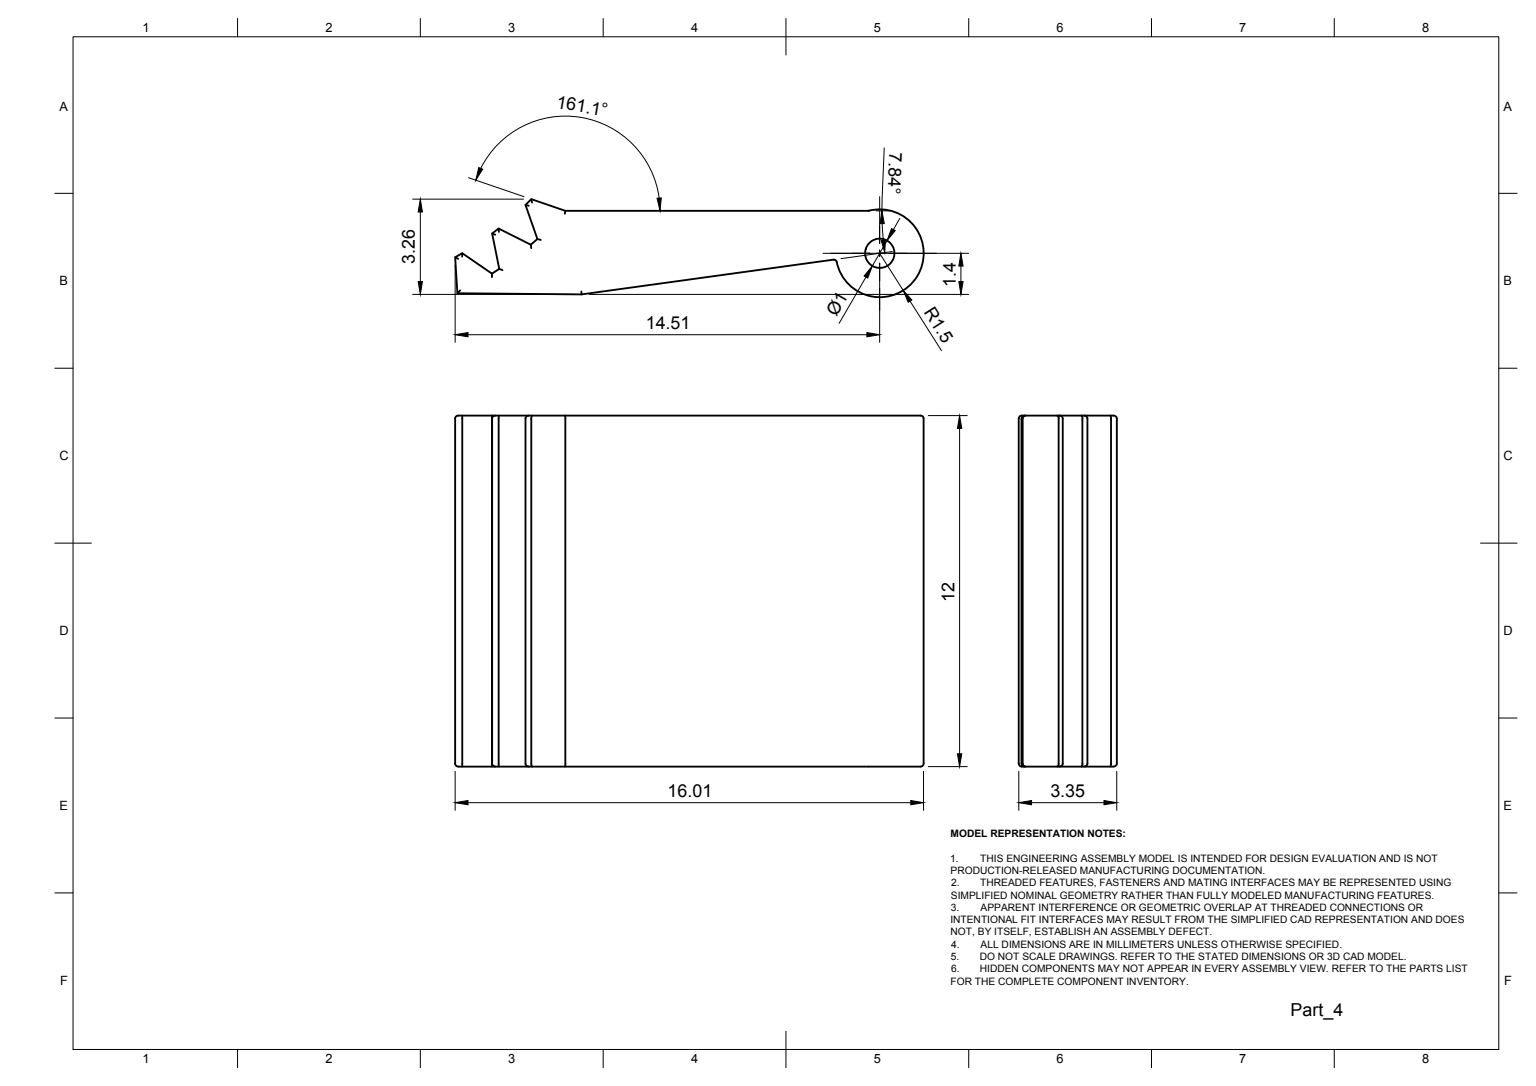
ISO-10303-21;
HEADER;
/* Generated by software containing ST-Developer
 * from STEP Tools, Inc. (www.steptools.com) 
 */

FILE_DESCRIPTION(
/* description */ ('STEP AP242 Edition 2'),
/* implementation_level */ '2;1');

FILE_NAME(
/* name */ 'Part_4.step',
/* time_stamp */ '2026-10-06T10:11:12-07:00',
/* author */ (''),
/* organization */ (''),
/* preprocessor_version */ 'ST-DEVELOPER v20.2',
/* originating_system */ 'Autodesk Translation Framework v15.15.0.0',
/* authorisation */ '');

FILE_SCHEMA (('AUTOMOTIVE_DESIGN { 1 0 10303 214 3 1 1 }'));
ENDSEC;

DATA;
#10=MECHANICAL_DESIGN_GEOMETRIC_PRESENTATION_REPRESENTATION('',(#1792),#54580);
#72=ELLIPSE('',#18845,0.000117970312899575,0.0001);
#73=ELLIPSE('',#18846,0.000120617936713865,0.0001);
#74=ELLIPSE('',#18848,0.000120617936713866,0.0001);
#75=ELLIPSE('',#18850,0.000120617936713866,0.0001);
#76=ELLIPSE('',#18851,0.000120617936713865,0.0001);
#77=ELLIPSE('',#18853,0.000117970312899575,0.0001);
#78=ELLIPSE('',#18855,0.000117970312899575,0.0001);
#79=ELLIPSE('',#18857,0.000117970312899574,0.0001);
#80=ELLIPSE('',#18859,0.000117970312899574,0.0001);
#81=ELLIPSE('',#18861,0.000117970312899575,0.0001);
#82=ELLIPSE('',#18863,0.000120617936713865,0.0001);
#83=ELLIPSE('',#18865,0.000117970312899575,0.0001);
#84=ELLIPSE('',#18867,0.000117970312899575,0.0001);
#85=ELLIPSE('',#18869,0.000120617936713865,0.0001);
#86=ELLIPSE('',#18871,0.000120617936713865,0.0001);
#87=ELLIPSE('',#18873,0.000136567519156022,0.0001);
#88=ELLIPSE('',#18875,0.000136567519156022,0.0001);
#89=ELLIPSE('',#18877,0.000120617936713865,0.0001);
#90=ELLIPSE('',#18879,0.000117970312899574,0.0001);
#91=ELLIPSE('',#18881,0.000100268099705458,0.0001);
#92=ELLIPSE('',#18883,0.000100268099705458,0.0001);
#93=ELLIPSE('',#18885,0.000117970312899574,0.0001);
#94=ELLIPSE('',#18887,0.000117970312899575,0.0001);
#95=ELLIPSE('',#18896,0.000117970312899575,0.0001);
#96=ELLIPSE('',#18898,0.000101375812252276,0.0001);
#97=ELLIPSE('',#18904,0.000101375812252276,0.0001);
#240=TOROIDAL_SURFACE('',#18899,0.0002,0.0001);
#241=TOROIDAL_SURFACE('',#18901,0.0002,0.0001);
#242=TOROIDAL_SURFACE('',#18907,0.0014,0.0001);
#243=TOROIDAL_SURFACE('',#18909,0.0014,0.0001);
#244=TOROIDAL_SURFACE('',#18913,0.0002,0.0001);
#245=TOROIDAL_SURFACE('',#18915,0.0002,0.0001);
#246=TOROIDAL_SURFACE('',#18918,0.0006,0.0001);
#247=TOROIDAL_SURFACE('',#18920,0.0006,0.0001);
#1748=SHAPE_REPRESENTATION_RELATIONSHIP('SRR','None',#54635,#1762);
#1762=ADVANCED_BREP_SHAPE_REPRESENTATION('',(#1806),#54571);
#1792=STYLED_ITEM('',(#54716),#1806);
#1806=MANIFOLD_SOLID_BREP('Body1',#17671);
#2101=LINE('',#47988,#2694);
#2102=LINE('',#47990,#2695);
#2103=LINE('',#47992,#2696);
#2104=LINE('',#47994,#2697);
#2105=LINE('',#47996,#2698);
#2106=LINE('',#47998,#2699);
#2107=LINE('',#48000,#2700);
#2108=LINE('',#48002,#2701);
#2109=LINE('',#48004,#2702);
#2110=LINE('',#48012,#2703);
#2111=LINE('',#48014,#2704);
#2112=LINE('',#48016,#2705);
#2113=LINE('',#48018,#2706);
#2114=LINE('',#48019,#2707);
#2115=LINE('',#48025,#2708);
#2116=LINE('',#48027,#2709);
#2117=LINE('',#48029,#2710);
#2118=LINE('',#48031,#2711);
#2119=LINE('',#48033,#2712);
#2120=LINE('',#48035,#2713);
#2121=LINE('',#48037,#2714);
#2122=LINE('',#48039,#2715);
#2123=LINE('',#48041,#2716);
#2124=LINE('',#48043,#2717);
#2125=LINE('',#48045,#2718);
#2126=LINE('',#48047,#2719);
#2127=LINE('',#48049,#2720);
#2128=LINE('',#48051,#2721);
#2129=LINE('',#48062,#2722);
#2130=LINE('',#48064,#2723);
#2131=LINE('',#48066,#2724);
#2132=LINE('',#48067,#2725);
#2133=LINE('',#48071,#2726);
#2134=LINE('',#48072,#2727);
#2135=LINE('',#48073,#2728);
#2136=LINE('',#48077,#2729);
#2137=LINE('',#48078,#2730);
#2138=LINE('',#48079,#2731);
#2139=LINE('',#48083,#2732);
#2140=LINE('',#48084,#2733);
#2141=LINE('',#48085,#2734);
#2142=LINE('',#48089,#2735);
#2143=LINE('',#48090,#2736);
#2144=LINE('',#48091,#2737);
#2145=LINE('',#48095,#2738);
#2146=LINE('',#48096,#2739);
#2147=LINE('',#48097,#2740);
#2148=LINE('',#48101,#2741);
#2149=LINE('',#48102,#2742);
#2150=LINE('',#48103,#2743);
#2151=LINE('',#48107,#2744);
#2152=LINE('',#48108,#2745);
#2153=LINE('',#48109,#2746);
#2154=LINE('',#48113,#2747);
#2155=LINE('',#48114,#2748);
#2156=LINE('',#48115,#2749);
#2157=LINE('',#48119,#2750);
#2158=LINE('',#48123,#2751);
#2159=LINE('',#48128,#2752);
#2160=LINE('',#48130,#2753);
#2161=LINE('',#48132,#2754);
#2162=LINE('',#48133,#2755);
#2163=LINE('',#48137,#2756);
#2164=LINE('',#48138,#2757);
#2165=LINE('',#48139,#2758);
#2166=LINE('',#48143,#2759);
#2167=LINE('',#48144,#2760);
#2168=LINE('',#48145,#2761);
#2169=LINE('',#48149,#2762);
#2170=LINE('',#48150,#2763);
#2171=LINE('',#48151,#2764);
#2172=LINE('',#48153,#2765);
#2173=LINE('',#48154,#2766);
#2174=LINE('',#48161,#2767);
#2694=VECTOR('',#21845,0.999999999999999);
#2695=VECTOR('',#21846,1.);
#2696=VECTOR('',#21847,1.);
#2697=VECTOR('',#21848,1.);
#2698=VECTOR('',#21849,1.);
#2699=VECTOR('',#21850,1.);
#2700=VECTOR('',#21851,1.);
#2701=VECTOR('',#21852,1.);
#2702=VECTOR('',#21853,1.);
#2703=VECTOR('',#21860,1.);
#2704=VECTOR('',#21861,1.);
#2705=VECTOR('',#21862,1.);
#2706=VECTOR('',#21863,1.);
#2707=VECTOR('',#21864,1.);
#2708=VECTOR('',#21869,1.);
#2709=VECTOR('',#21870,1.);
#2710=VECTOR('',#21871,1.);
#2711=VECTOR('',#21872,1.);
#2712=VECTOR('',#21873,1.);
#2713=VECTOR('',#21874,1.);
#2714=VECTOR('',#21875,1.);
#2715=VECTOR('',#21876,1.);
#2716=VECTOR('',#21877,0.999999999999999);
#2717=VECTOR('',#21878,1.);
#2718=VECTOR('',#21879,1.);
#2719=VECTOR('',#21880,1.);
#2720=VECTOR('',#21881,1.);
#2721=VECTOR('',#21882,1.);
#2722=VECTOR('',#21893,1.);
#2723=VECTOR('',#21894,1.);
#2724=VECTOR('',#21895,1.);
#2725=VECTOR('',#21896,1.);
#2726=VECTOR('',#21899,1.);
#2727=VECTOR('',#21900,1.);
#2728=VECTOR('',#21901,1.);
#2729=VECTOR('',#21904,1.);
#2730=VECTOR('',#21905,1.);
#2731=VECTOR('',#21906,1.);
#2732=VECTOR('',#21909,1.);
#2733=VECTOR('',#21910,0.999999999999999);
#2734=VECTOR('',#21911,0.999999999999999);
#2735=VECTOR('',#21914,1.);
#2736=VECTOR('',#21915,1.);
#2737=VECTOR('',#21916,1.);
#2738=VECTOR('',#21919,1.);
#2739=VECTOR('',#21920,1.);
#2740=VECTOR('',#21921,1.);
#2741=VECTOR('',#21924,1.);
#2742=VECTOR('',#21925,1.);
#2743=VECTOR('',#21926,1.);
#2744=VECTOR('',#21929,1.);
#2745=VECTOR('',#21930,1.);
#2746=VECTOR('',#21931,1.);
#2747=VECTOR('',#21934,1.);
#2748=VECTOR('',#21935,1.);
#2749=VECTOR('',#21936,1.);
#2750=VECTOR('',#21939,1.);
#2751=VECTOR('',#21942,1.);
#2752=VECTOR('',#21947,1.);
#2753=VECTOR('',#21948,1.);
#2754=VECTOR('',#21949,1.);
#2755=VECTOR('',#21950,1.);
#2756=VECTOR('',#21953,1.);
#2757=VECTOR('',#21954,1.);
#2758=VECTOR('',#21955,1.);
#2759=VECTOR('',#21958,1.);
#2760=VECTOR('',#21959,1.);
#2761=VECTOR('',#21960,1.);
#2762=VECTOR('',#21963,1.);
#2763=VECTOR('',#21964,1.);
#2764=VECTOR('',#21965,1.);
#2765=VECTOR('',#21968,1.);
#2766=VECTOR('',#21969,1.);
#2767=VECTOR('',#21976,0.0005);
#3329=CYLINDRICAL_SURFACE('',#18832,0.0015);
#3330=CYLINDRICAL_SURFACE('',#18840,0.0005);
#3331=CYLINDRICAL_SURFACE('',#18844,0.0001);
#3332=CYLINDRICAL_SURFACE('',#18847,0.0001);
#3333=CYLINDRICAL_SURFACE('',#18849,0.0001);
#3334=CYLINDRICAL_SURFACE('',#18852,0.0001);
#3335=CYLINDRICAL_SURFACE('',#18854,0.0001);
#3336=CYLINDRICAL_SURFACE('',#18856,0.0001);
#3337=CYLINDRICAL_SURFACE('',#18858,0.0001);
#3338=CYLINDRICAL_SURFACE('',#18860,0.0001);
#3339=CYLINDRICAL_SURFACE('',#18862,0.0001);
#3340=CYLINDRICAL_SURFACE('',#18864,0.0001);
#3341=CYLINDRICAL_SURFACE('',#18866,0.0001);
#3342=CYLINDRICAL_SURFACE('',#18868,0.0001);
#3343=CYLINDRICAL_SURFACE('',#18870,0.0001);
#3344=CYLINDRICAL_SURFACE('',#18872,0.0001);
#3345=CYLINDRICAL_SURFACE('',#18874,0.0001);
#3346=CYLINDRICAL_SURFACE('',#18876,0.0001);
#3347=CYLINDRICAL_SURFACE('',#18878,0.0001);
#3348=CYLINDRICAL_SURFACE('',#18880,0.0001);
#3349=CYLINDRICAL_SURFACE('',#18882,0.0001);
#3350=CYLINDRICAL_SURFACE('',#18884,0.0001);
#3351=CYLINDRICAL_SURFACE('',#18886,0.0001);
#3352=CYLINDRICAL_SURFACE('',#18888,0.0001);
#3353=CYLINDRICAL_SURFACE('',#18890,0.0001);
#3354=CYLINDRICAL_SURFACE('',#18893,0.0001);
#3355=CYLINDRICAL_SURFACE('',#18895,0.0001);
#3356=CYLINDRICAL_SURFACE('',#18897,0.0001);
#3357=CYLINDRICAL_SURFACE('',#18903,0.0001);
#3358=CYLINDRICAL_SURFACE('',#18905,0.0001);
#3359=CYLINDRICAL_SURFACE('',#18911,0.0001);
#3360=CYLINDRICAL_SURFACE('',#18917,0.0001);
#3506=FACE_BOUND('',#5205,.T.);
#3507=FACE_BOUND('',#5207,.T.);
#4169=FACE_OUTER_BOUND('',#5204,.T.);
#4170=FACE_OUTER_BOUND('',#5206,.T.);
#4171=FACE_OUTER_BOUND('',#5208,.T.);
#4172=FACE_OUTER_BOUND('',#5209,.T.);
#4173=FACE_OUTER_BOUND('',#5210,.T.);
#4174=FACE_OUTER_BOUND('',#5211,.T.);
#4175=FACE_OUTER_BOUND('',#5212,.T.);
#4176=FACE_OUTER_BOUND('',#5213,.T.);
#4177=FACE_OUTER_BOUND('',#5214,.T.);
#4178=FACE_OUTER_BOUND('',#5215,.T.);
#4179=FACE_OUTER_BOUND('',#5216,.T.);
#4180=FACE_OUTER_BOUND('',#5217,.T.);
#4181=FACE_OUTER_BOUND('',#5218,.T.);
#4182=FACE_OUTER_BOUND('',#5219,.T.);
#4183=FACE_OUTER_BOUND('',#5220,.T.);
#4184=FACE_OUTER_BOUND('',#5221,.T.);
#4185=FACE_OUTER_BOUND('',#5222,.T.);
#4186=FACE_OUTER_BOUND('',#5223,.T.);
#4187=FACE_OUTER_BOUND('',#5224,.T.);
#4188=FACE_OUTER_BOUND('',#5225,.T.);
#4189=FACE_OUTER_BOUND('',#5226,.T.);
#4190=FACE_OUTER_BOUND('',#5227,.T.);
#4191=FACE_OUTER_BOUND('',#5228,.T.);
#4192=FACE_OUTER_BOUND('',#5229,.T.);
#4193=FACE_OUTER_BOUND('',#5230,.T.);
#4194=FACE_OUTER_BOUND('',#5231,.T.);
#4195=FACE_OUTER_BOUND('',#5232,.T.);
#4196=FACE_OUTER_BOUND('',#5233,.T.);
#4197=FACE_OUTER_BOUND('',#5234,.T.);
#4198=FACE_OUTER_BOUND('',#5235,.T.);
#4199=FACE_OUTER_BOUND('',#5236,.T.);
#4200=FACE_OUTER_BOUND('',#5237,.T.);
#4201=FACE_OUTER_BOUND('',#5238,.T.);
#4202=FACE_OUTER_BOUND('',#5239,.T.);
#4203=FACE_OUTER_BOUND('',#5240,.T.);
#4204=FACE_OUTER_BOUND('',#5241,.T.);
#4205=FACE_OUTER_BOUND('',#5242,.T.);
#4206=FACE_OUTER_BOUND('',#5243,.T.);
#4207=FACE_OUTER_BOUND('',#5244,.T.);
#4208=FACE_OUTER_BOUND('',#5245,.T.);
#4209=FACE_OUTER_BOUND('',#5246,.T.);
#4210=FACE_OUTER_BOUND('',#5247,.T.);
#4211=FACE_OUTER_BOUND('',#5248,.T.);
#4212=FACE_OUTER_BOUND('',#5249,.T.);
#4213=FACE_OUTER_BOUND('',#5250,.T.);
#4214=FACE_OUTER_BOUND('',#5251,.T.);
#4215=FACE_OUTER_BOUND('',#5252,.T.);
#4216=FACE_OUTER_BOUND('',#5253,.T.);
#4217=FACE_OUTER_BOUND('',#5254,.T.);
#4218=FACE_OUTER_BOUND('',#5255,.T.);
#4219=FACE_OUTER_BOUND('',#5256,.T.);
#4220=FACE_OUTER_BOUND('',#5257,.T.);
#4221=FACE_OUTER_BOUND('',#5258,.T.);
#4222=FACE_OUTER_BOUND('',#5259,.T.);
#4223=FACE_OUTER_BOUND('',#5260,.T.);
#4224=FACE_OUTER_BOUND('',#5261,.T.);
#5204=EDGE_LOOP('',(#14741,#14742,#14743,#14744,#14745,#14746,#14747,#14748,
#14749,#14750,#14751,#14752,#14753,#14754,#14755,#14756,#14757));
#5205=EDGE_LOOP('',(#14758));
#5206=EDGE_LOOP('',(#14759,#14760,#14761,#14762,#14763,#14764,#14765,#14766,
#14767,#14768,#14769,#14770,#14771,#14772,#14773,#14774,#14775));
#5207=EDGE_LOOP('',(#14776));
#5208=EDGE_LOOP('',(#14777,#14778,#14779,#14780));
#5209=EDGE_LOOP('',(#14781,#14782,#14783,#14784));
#5210=EDGE_LOOP('',(#14785,#14786,#14787,#14788));
#5211=EDGE_LOOP('',(#14789,#14790,#14791,#14792));
#5212=EDGE_LOOP('',(#14793,#14794,#14795,#14796));
#5213=EDGE_LOOP('',(#14797,#14798,#14799,#14800));
#5214=EDGE_LOOP('',(#14801,#14802,#14803,#14804));
#5215=EDGE_LOOP('',(#14805,#14806,#14807,#14808));
#5216=EDGE_LOOP('',(#14809,#14810,#14811,#14812));
#5217=EDGE_LOOP('',(#14813,#14814,#14815,#14816));
#5218=EDGE_LOOP('',(#14817,#14818,#14819,#14820));
#5219=EDGE_LOOP('',(#14821,#14822,#14823,#14824));
#5220=EDGE_LOOP('',(#14825,#14826,#14827,#14828));
#5221=EDGE_LOOP('',(#14829,#14830,#14831,#14832));
#5222=EDGE_LOOP('',(#14833,#14834,#14835,#14836));
#5223=EDGE_LOOP('',(#14837,#14838,#14839,#14840,#14841));
#5224=EDGE_LOOP('',(#14842,#14843,#14844,#14845));
#5225=EDGE_LOOP('',(#14846,#14847,#14848,#14849));
#5226=EDGE_LOOP('',(#14850,#14851,#14852,#14853));
#5227=EDGE_LOOP('',(#14854,#14855,#14856,#14857));
#5228=EDGE_LOOP('',(#14858,#14859,#14860,#14861));
#5229=EDGE_LOOP('',(#14862,#14863,#14864,#14865));
#5230=EDGE_LOOP('',(#14866,#14867,#14868,#14869));
#5231=EDGE_LOOP('',(#14870,#14871,#14872,#14873));
#5232=EDGE_LOOP('',(#14874,#14875,#14876,#14877));
#5233=EDGE_LOOP('',(#14878,#14879,#14880,#14881));
#5234=EDGE_LOOP('',(#14882,#14883,#14884,#14885));
#5235=EDGE_LOOP('',(#14886,#14887,#14888,#14889));
#5236=EDGE_LOOP('',(#14890,#14891,#14892,#14893));
#5237=EDGE_LOOP('',(#14894,#14895,#14896,#14897));
#5238=EDGE_LOOP('',(#14898,#14899,#14900,#14901));
#5239=EDGE_LOOP('',(#14902,#14903,#14904,#14905));
#5240=EDGE_LOOP('',(#14906,#14907,#14908,#14909));
#5241=EDGE_LOOP('',(#14910,#14911,#14912,#14913));
#5242=EDGE_LOOP('',(#14914,#14915,#14916,#14917));
#5243=EDGE_LOOP('',(#14918,#14919,#14920,#14921));
#5244=EDGE_LOOP('',(#14922,#14923,#14924,#14925));
#5245=EDGE_LOOP('',(#14926,#14927,#14928,#14929));
#5246=EDGE_LOOP('',(#14930,#14931,#14932,#14933));
#5247=EDGE_LOOP('',(#14934,#14935,#14936,#14937));
#5248=EDGE_LOOP('',(#14938,#14939,#14940,#14941));
#5249=EDGE_LOOP('',(#14942,#14943,#14944,#14945));
#5250=EDGE_LOOP('',(#14946,#14947,#14948,#14949));
#5251=EDGE_LOOP('',(#14950,#14951,#14952,#14953));
#5252=EDGE_LOOP('',(#14954,#14955,#14956,#14957));
#5253=EDGE_LOOP('',(#14958,#14959,#14960,#14961));
#5254=EDGE_LOOP('',(#14962,#14963,#14964,#14965));
#5255=EDGE_LOOP('',(#14966,#14967,#14968,#14969));
#5256=EDGE_LOOP('',(#14970,#14971,#14972,#14973));
#5257=EDGE_LOOP('',(#14974,#14975,#14976,#14977));
#5258=EDGE_LOOP('',(#14978,#14979,#14980,#14981));
#5259=EDGE_LOOP('',(#14982,#14983,#14984,#14985));
#5260=EDGE_LOOP('',(#14986,#14987,#14988,#14989));
#5261=EDGE_LOOP('',(#14990,#14991,#14992,#14993,#14994));
#6159=CIRCLE('',#18814,0.0002);
#6160=CIRCLE('',#18815,0.0014);
#6161=CIRCLE('',#18816,0.0002);
#6162=CIRCLE('',#18817,0.0006);
#6163=CIRCLE('',#18819,0.0002);
#6164=CIRCLE('',#18820,0.0014);
#6165=CIRCLE('',#18821,0.0002);
#6166=CIRCLE('',#18822,0.0006);
#6167=CIRCLE('',#18833,0.0015);
#6168=CIRCLE('',#18834,0.0015);
#6169=CIRCLE('',#18841,0.0005);
#6170=CIRCLE('',#18842,0.0005);
#6171=CIRCLE('',#18843,0.0005);
#6172=CIRCLE('',#18889,0.0001);
#6173=CIRCLE('',#18891,0.0001);
#6174=CIRCLE('',#18892,0.0001);
#6175=CIRCLE('',#18894,0.0001);
#6176=CIRCLE('',#18900,0.0001);
#6177=CIRCLE('',#18902,0.0001);
#6178=CIRCLE('',#18906,0.0001);
#6179=CIRCLE('',#18908,0.0001);
#6180=CIRCLE('',#18910,0.0001);
#6181=CIRCLE('',#18912,0.0001);
#6182=CIRCLE('',#18914,0.0001);
#6183=CIRCLE('',#18916,0.0001);
#6184=CIRCLE('',#18919,0.0001);
#6185=CIRCLE('',#18921,0.0001);
#7772=VERTEX_POINT('',#47986);
#7773=VERTEX_POINT('',#47987);
#7774=VERTEX_POINT('',#47989);
#7775=VERTEX_POINT('',#47991);
#7776=VERTEX_POINT('',#47993);
#7777=VERTEX_POINT('',#47995);
#7778=VERTEX_POINT('',#47997);
#7779=VERTEX_POINT('',#47999);
#7780=VERTEX_POINT('',#48001);
#7781=VERTEX_POINT('',#48003);
#7782=VERTEX_POINT('',#48005);
#7783=VERTEX_POINT('',#48007);
#7784=VERTEX_POINT('',#48009);
#7785=VERTEX_POINT('',#48011);
#7786=VERTEX_POINT('',#48013);
#7787=VERTEX_POINT('',#48015);
#7788=VERTEX_POINT('',#48017);
#7789=VERTEX_POINT('',#48020);
#7790=VERTEX_POINT('',#48023);
#7791=VERTEX_POINT('',#48024);
#7792=VERTEX_POINT('',#48026);
#7793=VERTEX_POINT('',#48028);
#7794=VERTEX_POINT('',#48030);
#7795=VERTEX_POINT('',#48032);
#7796=VERTEX_POINT('',#48034);
#7797=VERTEX_POINT('',#48036);
#7798=VERTEX_POINT('',#48038);
#7799=VERTEX_POINT('',#48040);
#7800=VERTEX_POINT('',#48042);
#7801=VERTEX_POINT('',#48044);
#7802=VERTEX_POINT('',#48046);
#7803=VERTEX_POINT('',#48048);
#7804=VERTEX_POINT('',#48050);
#7805=VERTEX_POINT('',#48052);
#7806=VERTEX_POINT('',#48054);
#7807=VERTEX_POINT('',#48057);
#7808=VERTEX_POINT('',#48060);
#7809=VERTEX_POINT('',#48061);
#7810=VERTEX_POINT('',#48063);
#7811=VERTEX_POINT('',#48065);
#7812=VERTEX_POINT('',#48069);
#7813=VERTEX_POINT('',#48070);
#7814=VERTEX_POINT('',#48075);
#7815=VERTEX_POINT('',#48076);
#7816=VERTEX_POINT('',#48081);
#7817=VERTEX_POINT('',#48082);
#7818=VERTEX_POINT('',#48087);
#7819=VERTEX_POINT('',#48088);
#7820=VERTEX_POINT('',#48093);
#7821=VERTEX_POINT('',#48094);
#7822=VERTEX_POINT('',#48099);
#7823=VERTEX_POINT('',#48100);
#7824=VERTEX_POINT('',#48105);
#7825=VERTEX_POINT('',#48106);
#7826=VERTEX_POINT('',#48111);
#7827=VERTEX_POINT('',#48112);
#7828=VERTEX_POINT('',#48117);
#7829=VERTEX_POINT('',#48118);
#7830=VERTEX_POINT('',#48120);
#7831=VERTEX_POINT('',#48122);
#7832=VERTEX_POINT('',#48126);
#7833=VERTEX_POINT('',#48127);
#7834=VERTEX_POINT('',#48129);
#7835=VERTEX_POINT('',#48131);
#7836=VERTEX_POINT('',#48135);
#7837=VERTEX_POINT('',#48136);
#7838=VERTEX_POINT('',#48141);
#7839=VERTEX_POINT('',#48142);
#7840=VERTEX_POINT('',#48147);
#7841=VERTEX_POINT('',#48148);
#7842=VERTEX_POINT('',#48156);
#7843=VERTEX_POINT('',#48157);
#7844=VERTEX_POINT('',#48160);
#10162=EDGE_CURVE('',#7772,#7773,#2101,.F.);
#10163=EDGE_CURVE('',#7773,#7774,#2102,.F.);
#10164=EDGE_CURVE('',#7774,#7775,#2103,.F.);
#10165=EDGE_CURVE('',#7775,#7776,#2104,.F.);
#10166=EDGE_CURVE('',#7776,#7777,#2105,.F.);
#10167=EDGE_CURVE('',#7777,#7778,#2106,.F.);
#10168=EDGE_CURVE('',#7778,#7779,#2107,.F.);
#10169=EDGE_CURVE('',#7779,#7780,#2108,.F.);
#10170=EDGE_CURVE('',#7780,#7781,#2109,.F.);
#10171=EDGE_CURVE('',#7782,#7781,#6159,.T.);
#10172=EDGE_CURVE('',#7782,#7783,#6160,.T.);
#10173=EDGE_CURVE('',#7784,#7783,#6161,.T.);
#10174=EDGE_CURVE('',#7784,#7785,#2110,.F.);
#10175=EDGE_CURVE('',#7785,#7786,#2111,.F.);
#10176=EDGE_CURVE('',#7786,#7787,#2112,.F.);
#10177=EDGE_CURVE('',#7787,#7788,#2113,.F.);
#10178=EDGE_CURVE('',#7788,#7772,#2114,.F.);
#10179=EDGE_CURVE('',#7789,#7789,#6162,.F.);
#10180=EDGE_CURVE('',#7790,#7791,#2115,.T.);
#10181=EDGE_CURVE('',#7791,#7792,#2116,.T.);
#10182=EDGE_CURVE('',#7792,#7793,#2117,.T.);
#10183=EDGE_CURVE('',#7793,#7794,#2118,.T.);
#10184=EDGE_CURVE('',#7794,#7795,#2119,.T.);
#10185=EDGE_CURVE('',#7795,#7796,#2120,.T.);
#10186=EDGE_CURVE('',#7796,#7797,#2121,.T.);
#10187=EDGE_CURVE('',#7797,#7798,#2122,.T.);
#10188=EDGE_CURVE('',#7798,#7799,#2123,.T.);
#10189=EDGE_CURVE('',#7799,#7800,#2124,.T.);
#10190=EDGE_CURVE('',#7800,#7801,#2125,.T.);
#10191=EDGE_CURVE('',#7801,#7802,#2126,.T.);
#10192=EDGE_CURVE('',#7802,#7803,#2127,.T.);
#10193=EDGE_CURVE('',#7803,#7804,#2128,.T.);
#10194=EDGE_CURVE('',#7805,#7804,#6163,.T.);
#10195=EDGE_CURVE('',#7805,#7806,#6164,.T.);
#10196=EDGE_CURVE('',#7790,#7806,#6165,.T.);
#10197=EDGE_CURVE('',#7807,#7807,#6166,.F.);
#10198=EDGE_CURVE('',#7808,#7809,#2129,.T.);
#10199=EDGE_CURVE('',#7809,#7810,#2130,.F.);
#10200=EDGE_CURVE('',#7811,#7810,#2131,.T.);
#10201=EDGE_CURVE('',#7811,#7808,#2132,.T.);
#10202=EDGE_CURVE('',#7812,#7813,#2133,.T.);
#10203=EDGE_CURVE('',#7813,#7809,#2134,.F.);
#10204=EDGE_CURVE('',#7808,#7812,#2135,.T.);
#10205=EDGE_CURVE('',#7814,#7815,#2136,.T.);
#10206=EDGE_CURVE('',#7815,#7813,#2137,.F.);
#10207=EDGE_CURVE('',#7812,#7814,#2138,.T.);
#10208=EDGE_CURVE('',#7816,#7817,#2139,.T.);
#10209=EDGE_CURVE('',#7817,#7815,#2140,.F.);
#10210=EDGE_CURVE('',#7814,#7816,#2141,.T.);
#10211=EDGE_CURVE('',#7818,#7819,#2142,.T.);
#10212=EDGE_CURVE('',#7819,#7817,#2143,.F.);
#10213=EDGE_CURVE('',#7816,#7818,#2144,.T.);
#10214=EDGE_CURVE('',#7820,#7821,#2145,.T.);
#10215=EDGE_CURVE('',#7821,#7819,#2146,.F.);
#10216=EDGE_CURVE('',#7818,#7820,#2147,.T.);
#10217=EDGE_CURVE('',#7822,#7823,#2148,.T.);
#10218=EDGE_CURVE('',#7823,#7821,#2149,.F.);
#10219=EDGE_CURVE('',#7820,#7822,#2150,.T.);
#10220=EDGE_CURVE('',#7824,#7825,#2151,.T.);
#10221=EDGE_CURVE('',#7825,#7823,#2152,.F.);
#10222=EDGE_CURVE('',#7822,#7824,#2153,.T.);
#10223=EDGE_CURVE('',#7826,#7827,#2154,.F.);
#10224=EDGE_CURVE('',#7827,#7825,#2155,.F.);
#10225=EDGE_CURVE('',#7824,#7826,#2156,.T.);
#10226=EDGE_CURVE('',#7828,#7829,#2157,.T.);
#10227=EDGE_CURVE('',#7829,#7830,#6167,.F.);
#10228=EDGE_CURVE('',#7830,#7831,#2158,.F.);
#10229=EDGE_CURVE('',#7831,#7828,#6168,.F.);
#10230=EDGE_CURVE('',#7832,#7833,#2159,.T.);
#10231=EDGE_CURVE('',#7833,#7834,#2160,.F.);
#10232=EDGE_CURVE('',#7834,#7835,#2161,.T.);
#10233=EDGE_CURVE('',#7835,#7832,#2162,.T.);
#10234=EDGE_CURVE('',#7836,#7837,#2163,.T.);
#10235=EDGE_CURVE('',#7837,#7833,#2164,.F.);
#10236=EDGE_CURVE('',#7832,#7836,#2165,.T.);
#10237=EDGE_CURVE('',#7838,#7839,#2166,.T.);
#10238=EDGE_CURVE('',#7839,#7837,#2167,.F.);
#10239=EDGE_CURVE('',#7836,#7838,#2168,.T.);
#10240=EDGE_CURVE('',#7840,#7841,#2169,.T.);
#10241=EDGE_CURVE('',#7841,#7839,#2170,.F.);
#10242=EDGE_CURVE('',#7838,#7840,#2171,.T.);
#10243=EDGE_CURVE('',#7810,#7841,#2172,.F.);
#10244=EDGE_CURVE('',#7840,#7811,#2173,.T.);
#10245=EDGE_CURVE('',#7842,#7843,#6169,.T.);
#10246=EDGE_CURVE('',#7843,#7842,#6170,.T.);
#10247=EDGE_CURVE('',#7842,#7844,#2174,.T.);
#10248=EDGE_CURVE('',#7844,#7844,#6171,.T.);
#10249=EDGE_CURVE('',#7774,#7812,#72,.F.);
#10250=EDGE_CURVE('',#7814,#7773,#73,.T.);
#10251=EDGE_CURVE('',#7816,#7772,#74,.T.);
#10252=EDGE_CURVE('',#7799,#7817,#75,.T.);
#10253=EDGE_CURVE('',#7815,#7798,#76,.F.);
#10254=EDGE_CURVE('',#7813,#7797,#77,.F.);
#10255=EDGE_CURVE('',#7775,#7808,#78,.F.);
#10256=EDGE_CURVE('',#7818,#7788,#79,.T.);
#10257=EDGE_CURVE('',#7800,#7819,#80,.T.);
#10258=EDGE_CURVE('',#7809,#7796,#81,.F.);
#10259=EDGE_CURVE('',#7776,#7811,#82,.F.);
#10260=EDGE_CURVE('',#7820,#7787,#83,.T.);
#10261=EDGE_CURVE('',#7801,#7821,#84,.T.);
#10262=EDGE_CURVE('',#7810,#7795,#85,.F.);
#10263=EDGE_CURVE('',#7777,#7840,#86,.F.);
#10264=EDGE_CURVE('',#7822,#7786,#87,.T.);
#10265=EDGE_CURVE('',#7802,#7823,#88,.T.);
#10266=EDGE_CURVE('',#7841,#7794,#89,.F.);
#10267=EDGE_CURVE('',#7778,#7838,#90,.F.);
#10268=EDGE_CURVE('',#7824,#7785,#91,.T.);
#10269=EDGE_CURVE('',#7803,#7825,#92,.T.);
#10270=EDGE_CURVE('',#7839,#7793,#93,.F.);
#10271=EDGE_CURVE('',#7779,#7836,#94,.F.);
#10272=EDGE_CURVE('',#7826,#7784,#6172,.T.);
#10273=EDGE_CURVE('',#7827,#7830,#6173,.F.);
#10274=EDGE_CURVE('',#7831,#7826,#6174,.F.);
#10275=EDGE_CURVE('',#7804,#7827,#6175,.T.);
#10276=EDGE_CURVE('',#7837,#7792,#95,.F.);
#10277=EDGE_CURVE('',#7780,#7832,#96,.F.);
#10278=EDGE_CURVE('',#7831,#7783,#6176,.F.);
#10279=EDGE_CURVE('',#7805,#7830,#6177,.F.);
#10280=EDGE_CURVE('',#7833,#7791,#97,.F.);
#10281=EDGE_CURVE('',#7781,#7835,#6178,.T.);
#10282=EDGE_CURVE('',#7828,#7782,#6179,.T.);
#10283=EDGE_CURVE('',#7806,#7829,#6180,.T.);
#10284=EDGE_CURVE('',#7834,#7790,#6181,.T.);
#10285=EDGE_CURVE('',#7828,#7835,#6182,.T.);
#10286=EDGE_CURVE('',#7834,#7829,#6183,.T.);
#10287=EDGE_CURVE('',#7844,#7807,#6184,.T.);
#10288=EDGE_CURVE('',#7843,#7789,#6185,.T.);
#14741=ORIENTED_EDGE('',*,*,#10162,.T.);
#14742=ORIENTED_EDGE('',*,*,#10163,.T.);
#14743=ORIENTED_EDGE('',*,*,#10164,.T.);
#14744=ORIENTED_EDGE('',*,*,#10165,.T.);
#14745=ORIENTED_EDGE('',*,*,#10166,.T.);
#14746=ORIENTED_EDGE('',*,*,#10167,.T.);
#14747=ORIENTED_EDGE('',*,*,#10168,.T.);
#14748=ORIENTED_EDGE('',*,*,#10169,.T.);
#14749=ORIENTED_EDGE('',*,*,#10170,.T.);
#14750=ORIENTED_EDGE('',*,*,#10171,.F.);
#14751=ORIENTED_EDGE('',*,*,#10172,.T.);
#14752=ORIENTED_EDGE('',*,*,#10173,.F.);
#14753=ORIENTED_EDGE('',*,*,#10174,.T.);
#14754=ORIENTED_EDGE('',*,*,#10175,.T.);
#14755=ORIENTED_EDGE('',*,*,#10176,.T.);
#14756=ORIENTED_EDGE('',*,*,#10177,.T.);
#14757=ORIENTED_EDGE('',*,*,#10178,.T.);
#14758=ORIENTED_EDGE('',*,*,#10179,.T.);
#14759=ORIENTED_EDGE('',*,*,#10180,.T.);
#14760=ORIENTED_EDGE('',*,*,#10181,.T.);
#14761=ORIENTED_EDGE('',*,*,#10182,.T.);
#14762=ORIENTED_EDGE('',*,*,#10183,.T.);
#14763=ORIENTED_EDGE('',*,*,#10184,.T.);
#14764=ORIENTED_EDGE('',*,*,#10185,.T.);
#14765=ORIENTED_EDGE('',*,*,#10186,.T.);
#14766=ORIENTED_EDGE('',*,*,#10187,.T.);
#14767=ORIENTED_EDGE('',*,*,#10188,.T.);
#14768=ORIENTED_EDGE('',*,*,#10189,.T.);
#14769=ORIENTED_EDGE('',*,*,#10190,.T.);
#14770=ORIENTED_EDGE('',*,*,#10191,.T.);
#14771=ORIENTED_EDGE('',*,*,#10192,.T.);
#14772=ORIENTED_EDGE('',*,*,#10193,.T.);
#14773=ORIENTED_EDGE('',*,*,#10194,.F.);
#14774=ORIENTED_EDGE('',*,*,#10195,.T.);
#14775=ORIENTED_EDGE('',*,*,#10196,.F.);
#14776=ORIENTED_EDGE('',*,*,#10197,.T.);
#14777=ORIENTED_EDGE('',*,*,#10198,.T.);
#14778=ORIENTED_EDGE('',*,*,#10199,.T.);
#14779=ORIENTED_EDGE('',*,*,#10200,.F.);
#14780=ORIENTED_EDGE('',*,*,#10201,.T.);
#14781=ORIENTED_EDGE('',*,*,#10202,.T.);
#14782=ORIENTED_EDGE('',*,*,#10203,.T.);
#14783=ORIENTED_EDGE('',*,*,#10198,.F.);
#14784=ORIENTED_EDGE('',*,*,#10204,.T.);
#14785=ORIENTED_EDGE('',*,*,#10205,.T.);
#14786=ORIENTED_EDGE('',*,*,#10206,.T.);
#14787=ORIENTED_EDGE('',*,*,#10202,.F.);
#14788=ORIENTED_EDGE('',*,*,#10207,.T.);
#14789=ORIENTED_EDGE('',*,*,#10208,.T.);
#14790=ORIENTED_EDGE('',*,*,#10209,.T.);
#14791=ORIENTED_EDGE('',*,*,#10205,.F.);
#14792=ORIENTED_EDGE('',*,*,#10210,.T.);
#14793=ORIENTED_EDGE('',*,*,#10211,.T.);
#14794=ORIENTED_EDGE('',*,*,#10212,.T.);
#14795=ORIENTED_EDGE('',*,*,#10208,.F.);
#14796=ORIENTED_EDGE('',*,*,#10213,.T.);
#14797=ORIENTED_EDGE('',*,*,#10214,.T.);
#14798=ORIENTED_EDGE('',*,*,#10215,.T.);
#14799=ORIENTED_EDGE('',*,*,#10211,.F.);
#14800=ORIENTED_EDGE('',*,*,#10216,.T.);
#14801=ORIENTED_EDGE('',*,*,#10217,.T.);
#14802=ORIENTED_EDGE('',*,*,#10218,.T.);
#14803=ORIENTED_EDGE('',*,*,#10214,.F.);
#14804=ORIENTED_EDGE('',*,*,#10219,.T.);
#14805=ORIENTED_EDGE('',*,*,#10220,.T.);
#14806=ORIENTED_EDGE('',*,*,#10221,.T.);
#14807=ORIENTED_EDGE('',*,*,#10217,.F.);
#14808=ORIENTED_EDGE('',*,*,#10222,.T.);
#14809=ORIENTED_EDGE('',*,*,#10223,.T.);
#14810=ORIENTED_EDGE('',*,*,#10224,.T.);
#14811=ORIENTED_EDGE('',*,*,#10220,.F.);
#14812=ORIENTED_EDGE('',*,*,#10225,.T.);
#14813=ORIENTED_EDGE('',*,*,#10226,.T.);
#14814=ORIENTED_EDGE('',*,*,#10227,.T.);
#14815=ORIENTED_EDGE('',*,*,#10228,.T.);
#14816=ORIENTED_EDGE('',*,*,#10229,.T.);
#14817=ORIENTED_EDGE('',*,*,#10230,.T.);
#14818=ORIENTED_EDGE('',*,*,#10231,.T.);
#14819=ORIENTED_EDGE('',*,*,#10232,.T.);
#14820=ORIENTED_EDGE('',*,*,#10233,.T.);
#14821=ORIENTED_EDGE('',*,*,#10234,.T.);
#14822=ORIENTED_EDGE('',*,*,#10235,.T.);
#14823=ORIENTED_EDGE('',*,*,#10230,.F.);
#14824=ORIENTED_EDGE('',*,*,#10236,.T.);
#14825=ORIENTED_EDGE('',*,*,#10237,.T.);
#14826=ORIENTED_EDGE('',*,*,#10238,.T.);
#14827=ORIENTED_EDGE('',*,*,#10234,.F.);
#14828=ORIENTED_EDGE('',*,*,#10239,.T.);
#14829=ORIENTED_EDGE('',*,*,#10240,.T.);
#14830=ORIENTED_EDGE('',*,*,#10241,.T.);
#14831=ORIENTED_EDGE('',*,*,#10237,.F.);
#14832=ORIENTED_EDGE('',*,*,#10242,.T.);
#14833=ORIENTED_EDGE('',*,*,#10200,.T.);
#14834=ORIENTED_EDGE('',*,*,#10243,.T.);
#14835=ORIENTED_EDGE('',*,*,#10240,.F.);
#14836=ORIENTED_EDGE('',*,*,#10244,.T.);
#14837=ORIENTED_EDGE('',*,*,#10245,.T.);
#14838=ORIENTED_EDGE('',*,*,#10246,.T.);
#14839=ORIENTED_EDGE('',*,*,#10247,.T.);
#14840=ORIENTED_EDGE('',*,*,#10248,.T.);
#14841=ORIENTED_EDGE('',*,*,#10247,.F.);
#14842=ORIENTED_EDGE('',*,*,#10249,.F.);
#14843=ORIENTED_EDGE('',*,*,#10163,.F.);
#14844=ORIENTED_EDGE('',*,*,#10250,.F.);
#14845=ORIENTED_EDGE('',*,*,#10207,.F.);
#14846=ORIENTED_EDGE('',*,*,#10250,.T.);
#14847=ORIENTED_EDGE('',*,*,#10162,.F.);
#14848=ORIENTED_EDGE('',*,*,#10251,.F.);
#14849=ORIENTED_EDGE('',*,*,#10210,.F.);
#14850=ORIENTED_EDGE('',*,*,#10252,.F.);
#14851=ORIENTED_EDGE('',*,*,#10188,.F.);
#14852=ORIENTED_EDGE('',*,*,#10253,.F.);
#14853=ORIENTED_EDGE('',*,*,#10209,.F.);
#14854=ORIENTED_EDGE('',*,*,#10253,.T.);
#14855=ORIENTED_EDGE('',*,*,#10187,.F.);
#14856=ORIENTED_EDGE('',*,*,#10254,.F.);
#14857=ORIENTED_EDGE('',*,*,#10206,.F.);
#14858=ORIENTED_EDGE('',*,*,#10249,.T.);
#14859=ORIENTED_EDGE('',*,*,#10204,.F.);
#14860=ORIENTED_EDGE('',*,*,#10255,.F.);
#14861=ORIENTED_EDGE('',*,*,#10164,.F.);
#14862=ORIENTED_EDGE('',*,*,#10251,.T.);
#14863=ORIENTED_EDGE('',*,*,#10178,.F.);
#14864=ORIENTED_EDGE('',*,*,#10256,.F.);
#14865=ORIENTED_EDGE('',*,*,#10213,.F.);
#14866=ORIENTED_EDGE('',*,*,#10252,.T.);
#14867=ORIENTED_EDGE('',*,*,#10212,.F.);
#14868=ORIENTED_EDGE('',*,*,#10257,.F.);
#14869=ORIENTED_EDGE('',*,*,#10189,.F.);
#14870=ORIENTED_EDGE('',*,*,#10254,.T.);
#14871=ORIENTED_EDGE('',*,*,#10186,.F.);
#14872=ORIENTED_EDGE('',*,*,#10258,.F.);
#14873=ORIENTED_EDGE('',*,*,#10203,.F.);
#14874=ORIENTED_EDGE('',*,*,#10255,.T.);
#14875=ORIENTED_EDGE('',*,*,#10201,.F.);
#14876=ORIENTED_EDGE('',*,*,#10259,.F.);
#14877=ORIENTED_EDGE('',*,*,#10165,.F.);
#14878=ORIENTED_EDGE('',*,*,#10256,.T.);
#14879=ORIENTED_EDGE('',*,*,#10177,.F.);
#14880=ORIENTED_EDGE('',*,*,#10260,.F.);
#14881=ORIENTED_EDGE('',*,*,#10216,.F.);
#14882=ORIENTED_EDGE('',*,*,#10257,.T.);
#14883=ORIENTED_EDGE('',*,*,#10215,.F.);
#14884=ORIENTED_EDGE('',*,*,#10261,.F.);
#14885=ORIENTED_EDGE('',*,*,#10190,.F.);
#14886=ORIENTED_EDGE('',*,*,#10258,.T.);
#14887=ORIENTED_EDGE('',*,*,#10185,.F.);
#14888=ORIENTED_EDGE('',*,*,#10262,.F.);
#14889=ORIENTED_EDGE('',*,*,#10199,.F.);
#14890=ORIENTED_EDGE('',*,*,#10259,.T.);
#14891=ORIENTED_EDGE('',*,*,#10244,.F.);
#14892=ORIENTED_EDGE('',*,*,#10263,.F.);
#14893=ORIENTED_EDGE('',*,*,#10166,.F.);
#14894=ORIENTED_EDGE('',*,*,#10260,.T.);
#14895=ORIENTED_EDGE('',*,*,#10176,.F.);
#14896=ORIENTED_EDGE('',*,*,#10264,.F.);
#14897=ORIENTED_EDGE('',*,*,#10219,.F.);
#14898=ORIENTED_EDGE('',*,*,#10261,.T.);
#14899=ORIENTED_EDGE('',*,*,#10218,.F.);
#14900=ORIENTED_EDGE('',*,*,#10265,.F.);
#14901=ORIENTED_EDGE('',*,*,#10191,.F.);
#14902=ORIENTED_EDGE('',*,*,#10262,.T.);
#14903=ORIENTED_EDGE('',*,*,#10184,.F.);
#14904=ORIENTED_EDGE('',*,*,#10266,.F.);
#14905=ORIENTED_EDGE('',*,*,#10243,.F.);
#14906=ORIENTED_EDGE('',*,*,#10263,.T.);
#14907=ORIENTED_EDGE('',*,*,#10242,.F.);
#14908=ORIENTED_EDGE('',*,*,#10267,.F.);
#14909=ORIENTED_EDGE('',*,*,#10167,.F.);
#14910=ORIENTED_EDGE('',*,*,#10264,.T.);
#14911=ORIENTED_EDGE('',*,*,#10175,.F.);
#14912=ORIENTED_EDGE('',*,*,#10268,.F.);
#14913=ORIENTED_EDGE('',*,*,#10222,.F.);
#14914=ORIENTED_EDGE('',*,*,#10265,.T.);
#14915=ORIENTED_EDGE('',*,*,#10221,.F.);
#14916=ORIENTED_EDGE('',*,*,#10269,.F.);
#14917=ORIENTED_EDGE('',*,*,#10192,.F.);
#14918=ORIENTED_EDGE('',*,*,#10266,.T.);
#14919=ORIENTED_EDGE('',*,*,#10183,.F.);
#14920=ORIENTED_EDGE('',*,*,#10270,.F.);
#14921=ORIENTED_EDGE('',*,*,#10241,.F.);
#14922=ORIENTED_EDGE('',*,*,#10267,.T.);
#14923=ORIENTED_EDGE('',*,*,#10239,.F.);
#14924=ORIENTED_EDGE('',*,*,#10271,.F.);
#14925=ORIENTED_EDGE('',*,*,#10168,.F.);
#14926=ORIENTED_EDGE('',*,*,#10268,.T.);
#14927=ORIENTED_EDGE('',*,*,#10174,.F.);
#14928=ORIENTED_EDGE('',*,*,#10272,.F.);
#14929=ORIENTED_EDGE('',*,*,#10225,.F.);
#14930=ORIENTED_EDGE('',*,*,#10273,.F.);
#14931=ORIENTED_EDGE('',*,*,#10223,.F.);
#14932=ORIENTED_EDGE('',*,*,#10274,.F.);
#14933=ORIENTED_EDGE('',*,*,#10228,.F.);
#14934=ORIENTED_EDGE('',*,*,#10269,.T.);
#14935=ORIENTED_EDGE('',*,*,#10224,.F.);
#14936=ORIENTED_EDGE('',*,*,#10275,.F.);
#14937=ORIENTED_EDGE('',*,*,#10193,.F.);
#14938=ORIENTED_EDGE('',*,*,#10270,.T.);
#14939=ORIENTED_EDGE('',*,*,#10182,.F.);
#14940=ORIENTED_EDGE('',*,*,#10276,.F.);
#14941=ORIENTED_EDGE('',*,*,#10238,.F.);
#14942=ORIENTED_EDGE('',*,*,#10271,.T.);
#14943=ORIENTED_EDGE('',*,*,#10236,.F.);
#14944=ORIENTED_EDGE('',*,*,#10277,.F.);
#14945=ORIENTED_EDGE('',*,*,#10169,.F.);
#14946=ORIENTED_EDGE('',*,*,#10272,.T.);
#14947=ORIENTED_EDGE('',*,*,#10173,.T.);
#14948=ORIENTED_EDGE('',*,*,#10278,.F.);
#14949=ORIENTED_EDGE('',*,*,#10274,.T.);
#14950=ORIENTED_EDGE('',*,*,#10275,.T.);
#14951=ORIENTED_EDGE('',*,*,#10273,.T.);
#14952=ORIENTED_EDGE('',*,*,#10279,.F.);
#14953=ORIENTED_EDGE('',*,*,#10194,.T.);
#14954=ORIENTED_EDGE('',*,*,#10276,.T.);
#14955=ORIENTED_EDGE('',*,*,#10181,.F.);
#14956=ORIENTED_EDGE('',*,*,#10280,.F.);
#14957=ORIENTED_EDGE('',*,*,#10235,.F.);
#14958=ORIENTED_EDGE('',*,*,#10277,.T.);
#14959=ORIENTED_EDGE('',*,*,#10233,.F.);
#14960=ORIENTED_EDGE('',*,*,#10281,.F.);
#14961=ORIENTED_EDGE('',*,*,#10170,.F.);
#14962=ORIENTED_EDGE('',*,*,#10278,.T.);
#14963=ORIENTED_EDGE('',*,*,#10172,.F.);
#14964=ORIENTED_EDGE('',*,*,#10282,.F.);
#14965=ORIENTED_EDGE('',*,*,#10229,.F.);
#14966=ORIENTED_EDGE('',*,*,#10279,.T.);
#14967=ORIENTED_EDGE('',*,*,#10227,.F.);
#14968=ORIENTED_EDGE('',*,*,#10283,.F.);
#14969=ORIENTED_EDGE('',*,*,#10195,.F.);
#14970=ORIENTED_EDGE('',*,*,#10280,.T.);
#14971=ORIENTED_EDGE('',*,*,#10180,.F.);
#14972=ORIENTED_EDGE('',*,*,#10284,.F.);
#14973=ORIENTED_EDGE('',*,*,#10231,.F.);
#14974=ORIENTED_EDGE('',*,*,#10171,.T.);
#14975=ORIENTED_EDGE('',*,*,#10281,.T.);
#14976=ORIENTED_EDGE('',*,*,#10285,.F.);
#14977=ORIENTED_EDGE('',*,*,#10282,.T.);
#14978=ORIENTED_EDGE('',*,*,#10196,.T.);
#14979=ORIENTED_EDGE('',*,*,#10283,.T.);
#14980=ORIENTED_EDGE('',*,*,#10286,.F.);
#14981=ORIENTED_EDGE('',*,*,#10284,.T.);
#14982=ORIENTED_EDGE('',*,*,#10285,.T.);
#14983=ORIENTED_EDGE('',*,*,#10232,.F.);
#14984=ORIENTED_EDGE('',*,*,#10286,.T.);
#14985=ORIENTED_EDGE('',*,*,#10226,.F.);
#14986=ORIENTED_EDGE('',*,*,#10248,.F.);
#14987=ORIENTED_EDGE('',*,*,#10287,.T.);
#14988=ORIENTED_EDGE('',*,*,#10197,.F.);
#14989=ORIENTED_EDGE('',*,*,#10287,.F.);
#14990=ORIENTED_EDGE('',*,*,#10245,.F.);
#14991=ORIENTED_EDGE('',*,*,#10246,.F.);
#14992=ORIENTED_EDGE('',*,*,#10288,.T.);
#14993=ORIENTED_EDGE('',*,*,#10179,.F.);
#14994=ORIENTED_EDGE('',*,*,#10288,.F.);
#16575=PLANE('',#18813);
#16576=PLANE('',#18818);
#16577=PLANE('',#18823);
#16578=PLANE('',#18824);
#16579=PLANE('',#18825);
#16580=PLANE('',#18826);
#16581=PLANE('',#18827);
#16582=PLANE('',#18828);
#16583=PLANE('',#18829);
#16584=PLANE('',#18830);
#16585=PLANE('',#18831);
#16586=PLANE('',#18835);
#16587=PLANE('',#18836);
#16588=PLANE('',#18837);
#16589=PLANE('',#18838);
#16590=PLANE('',#18839);
#17285=ADVANCED_FACE('',(#4169,#3506),#16575,.T.);
#17286=ADVANCED_FACE('',(#4170,#3507),#16576,.T.);
#17287=ADVANCED_FACE('',(#4171),#16577,.T.);
#17288=ADVANCED_FACE('',(#4172),#16578,.T.);
#17289=ADVANCED_FACE('',(#4173),#16579,.T.);
#17290=ADVANCED_FACE('',(#4174),#16580,.T.);
#17291=ADVANCED_FACE('',(#4175),#16581,.T.);
#17292=ADVANCED_FACE('',(#4176),#16582,.T.);
#17293=ADVANCED_FACE('',(#4177),#16583,.T.);
#17294=ADVANCED_FACE('',(#4178),#16584,.T.);
#17295=ADVANCED_FACE('',(#4179),#16585,.T.);
#17296=ADVANCED_FACE('',(#4180),#3329,.T.);
#17297=ADVANCED_FACE('',(#4181),#16586,.T.);
#17298=ADVANCED_FACE('',(#4182),#16587,.T.);
#17299=ADVANCED_FACE('',(#4183),#16588,.T.);
#17300=ADVANCED_FACE('',(#4184),#16589,.T.);
#17301=ADVANCED_FACE('',(#4185),#16590,.T.);
#17302=ADVANCED_FACE('',(#4186),#3330,.F.);
#17303=ADVANCED_FACE('',(#4187),#3331,.T.);
#17304=ADVANCED_FACE('',(#4188),#3332,.T.);
#17305=ADVANCED_FACE('',(#4189),#3333,.T.);
#17306=ADVANCED_FACE('',(#4190),#3334,.T.);
#17307=ADVANCED_FACE('',(#4191),#3335,.T.);
#17308=ADVANCED_FACE('',(#4192),#3336,.T.);
#17309=ADVANCED_FACE('',(#4193),#3337,.T.);
#17310=ADVANCED_FACE('',(#4194),#3338,.T.);
#17311=ADVANCED_FACE('',(#4195),#3339,.T.);
#17312=ADVANCED_FACE('',(#4196),#3340,.T.);
#17313=ADVANCED_FACE('',(#4197),#3341,.T.);
#17314=ADVANCED_FACE('',(#4198),#3342,.T.);
#17315=ADVANCED_FACE('',(#4199),#3343,.T.);
#17316=ADVANCED_FACE('',(#4200),#3344,.T.);
#17317=ADVANCED_FACE('',(#4201),#3345,.T.);
#17318=ADVANCED_FACE('',(#4202),#3346,.T.);
#17319=ADVANCED_FACE('',(#4203),#3347,.T.);
#17320=ADVANCED_FACE('',(#4204),#3348,.T.);
#17321=ADVANCED_FACE('',(#4205),#3349,.T.);
#17322=ADVANCED_FACE('',(#4206),#3350,.T.);
#17323=ADVANCED_FACE('',(#4207),#3351,.T.);
#17324=ADVANCED_FACE('',(#4208),#3352,.T.);
#17325=ADVANCED_FACE('',(#4209),#3353,.F.);
#17326=ADVANCED_FACE('',(#4210),#3354,.T.);
#17327=ADVANCED_FACE('',(#4211),#3355,.T.);
#17328=ADVANCED_FACE('',(#4212),#3356,.T.);
#17329=ADVANCED_FACE('',(#4213),#240,.T.);
#17330=ADVANCED_FACE('',(#4214),#241,.T.);
#17331=ADVANCED_FACE('',(#4215),#3357,.T.);
#17332=ADVANCED_FACE('',(#4216),#3358,.T.);
#17333=ADVANCED_FACE('',(#4217),#242,.T.);
#17334=ADVANCED_FACE('',(#4218),#243,.T.);
#17335=ADVANCED_FACE('',(#4219),#3359,.T.);
#17336=ADVANCED_FACE('',(#4220),#244,.T.);
#17337=ADVANCED_FACE('',(#4221),#245,.T.);
#17338=ADVANCED_FACE('',(#4222),#3360,.F.);
#17339=ADVANCED_FACE('',(#4223),#246,.T.);
#17340=ADVANCED_FACE('',(#4224),#247,.T.);
#17671=CLOSED_SHELL('',(#17285,#17286,#17287,#17288,#17289,#17290,#17291,
#17292,#17293,#17294,#17295,#17296,#17297,#17298,#17299,#17300,#17301,#17302,
#17303,#17304,#17305,#17306,#17307,#17308,#17309,#17310,#17311,#17312,#17313,
#17314,#17315,#17316,#17317,#17318,#17319,#17320,#17321,#17322,#17323,#17324,
#17325,#17326,#17327,#17328,#17329,#17330,#17331,#17332,#17333,#17334,#17335,
#17336,#17337,#17338,#17339,#17340));
#18812=AXIS2_PLACEMENT_3D('',#47984,#21841,#21842);
#18813=AXIS2_PLACEMENT_3D('',#47985,#21843,#21844);
#18814=AXIS2_PLACEMENT_3D('',#48006,#21854,#21855);
#18815=AXIS2_PLACEMENT_3D('',#48008,#21856,#21857);
#18816=AXIS2_PLACEMENT_3D('',#48010,#21858,#21859);
#18817=AXIS2_PLACEMENT_3D('',#48021,#21865,#21866);
#18818=AXIS2_PLACEMENT_3D('',#48022,#21867,#21868);
#18819=AXIS2_PLACEMENT_3D('',#48053,#21883,#21884);
#18820=AXIS2_PLACEMENT_3D('',#48055,#21885,#21886);
#18821=AXIS2_PLACEMENT_3D('',#48056,#21887,#21888);
#18822=AXIS2_PLACEMENT_3D('',#48058,#21889,#21890);
#18823=AXIS2_PLACEMENT_3D('',#48059,#21891,#21892);
#18824=AXIS2_PLACEMENT_3D('',#48068,#21897,#21898);
#18825=AXIS2_PLACEMENT_3D('',#48074,#21902,#21903);
#18826=AXIS2_PLACEMENT_3D('',#48080,#21907,#21908);
#18827=AXIS2_PLACEMENT_3D('',#48086,#21912,#21913);
#18828=AXIS2_PLACEMENT_3D('',#48092,#21917,#21918);
#18829=AXIS2_PLACEMENT_3D('',#48098,#21922,#21923);
#18830=AXIS2_PLACEMENT_3D('',#48104,#21927,#21928);
#18831=AXIS2_PLACEMENT_3D('',#48110,#21932,#21933);
#18832=AXIS2_PLACEMENT_3D('',#48116,#21937,#21938);
#18833=AXIS2_PLACEMENT_3D('',#48121,#21940,#21941);
#18834=AXIS2_PLACEMENT_3D('',#48124,#21943,#21944);
#18835=AXIS2_PLACEMENT_3D('',#48125,#21945,#21946);
#18836=AXIS2_PLACEMENT_3D('',#48134,#21951,#21952);
#18837=AXIS2_PLACEMENT_3D('',#48140,#21956,#21957);
#18838=AXIS2_PLACEMENT_3D('',#48146,#21961,#21962);
#18839=AXIS2_PLACEMENT_3D('',#48152,#21966,#21967);
#18840=AXIS2_PLACEMENT_3D('',#48155,#21970,#21971);
#18841=AXIS2_PLACEMENT_3D('',#48158,#21972,#21973);
#18842=AXIS2_PLACEMENT_3D('',#48159,#21974,#21975);
#18843=AXIS2_PLACEMENT_3D('',#48162,#21977,#21978);
#18844=AXIS2_PLACEMENT_3D('',#48163,#21979,#21980);
#18845=AXIS2_PLACEMENT_3D('',#48164,#21981,#21982);
#18846=AXIS2_PLACEMENT_3D('',#48165,#21983,#21984);
#18847=AXIS2_PLACEMENT_3D('',#48166,#21985,#21986);
#18848=AXIS2_PLACEMENT_3D('',#48167,#21987,#21988);
#18849=AXIS2_PLACEMENT_3D('',#48168,#21989,#21990);
#18850=AXIS2_PLACEMENT_3D('',#48169,#21991,#21992);
#18851=AXIS2_PLACEMENT_3D('',#48170,#21993,#21994);
#18852=AXIS2_PLACEMENT_3D('',#48171,#21995,#21996);
#18853=AXIS2_PLACEMENT_3D('',#48172,#21997,#21998);
#18854=AXIS2_PLACEMENT_3D('',#48173,#21999,#22000);
#18855=AXIS2_PLACEMENT_3D('',#48174,#22001,#22002);
#18856=AXIS2_PLACEMENT_3D('',#48175,#22003,#22004);
#18857=AXIS2_PLACEMENT_3D('',#48176,#22005,#22006);
#18858=AXIS2_PLACEMENT_3D('',#48177,#22007,#22008);
#18859=AXIS2_PLACEMENT_3D('',#48178,#22009,#22010);
#18860=AXIS2_PLACEMENT_3D('',#48179,#22011,#22012);
#18861=AXIS2_PLACEMENT_3D('',#48180,#22013,#22014);
#18862=AXIS2_PLACEMENT_3D('',#48181,#22015,#22016);
#18863=AXIS2_PLACEMENT_3D('',#48182,#22017,#22018);
#18864=AXIS2_PLACEMENT_3D('',#48183,#22019,#22020);
#18865=AXIS2_PLACEMENT_3D('',#48184,#22021,#22022);
#18866=AXIS2_PLACEMENT_3D('',#48185,#22023,#22024);
#18867=AXIS2_PLACEMENT_3D('',#48186,#22025,#22026);
#18868=AXIS2_PLACEMENT_3D('',#48187,#22027,#22028);
#18869=AXIS2_PLACEMENT_3D('',#48188,#22029,#22030);
#18870=AXIS2_PLACEMENT_3D('',#48189,#22031,#22032);
#18871=AXIS2_PLACEMENT_3D('',#48190,#22033,#22034);
#18872=AXIS2_PLACEMENT_3D('',#48191,#22035,#22036);
#18873=AXIS2_PLACEMENT_3D('',#48192,#22037,#22038);
#18874=AXIS2_PLACEMENT_3D('',#48193,#22039,#22040);
#18875=AXIS2_PLACEMENT_3D('',#48194,#22041,#22042);
#18876=AXIS2_PLACEMENT_3D('',#48195,#22043,#22044);
#18877=AXIS2_PLACEMENT_3D('',#48196,#22045,#22046);
#18878=AXIS2_PLACEMENT_3D('',#48197,#22047,#22048);
#18879=AXIS2_PLACEMENT_3D('',#48198,#22049,#22050);
#18880=AXIS2_PLACEMENT_3D('',#48199,#22051,#22052);
#18881=AXIS2_PLACEMENT_3D('',#48200,#22053,#22054);
#18882=AXIS2_PLACEMENT_3D('',#48201,#22055,#22056);
#18883=AXIS2_PLACEMENT_3D('',#48202,#22057,#22058);
#18884=AXIS2_PLACEMENT_3D('',#48203,#22059,#22060);
#18885=AXIS2_PLACEMENT_3D('',#48204,#22061,#22062);
#18886=AXIS2_PLACEMENT_3D('',#48205,#22063,#22064);
#18887=AXIS2_PLACEMENT_3D('',#48206,#22065,#22066);
#18888=AXIS2_PLACEMENT_3D('',#48207,#22067,#22068);
#18889=AXIS2_PLACEMENT_3D('',#48208,#22069,#22070);
#18890=AXIS2_PLACEMENT_3D('',#48209,#22071,#22072);
#18891=AXIS2_PLACEMENT_3D('',#48210,#22073,#22074);
#18892=AXIS2_PLACEMENT_3D('',#48211,#22075,#22076);
#18893=AXIS2_PLACEMENT_3D('',#48212,#22077,#22078);
#18894=AXIS2_PLACEMENT_3D('',#48213,#22079,#22080);
#18895=AXIS2_PLACEMENT_3D('',#48214,#22081,#22082);
#18896=AXIS2_PLACEMENT_3D('',#48215,#22083,#22084);
#18897=AXIS2_PLACEMENT_3D('',#48216,#22085,#22086);
#18898=AXIS2_PLACEMENT_3D('',#48217,#22087,#22088);
#18899=AXIS2_PLACEMENT_3D('',#48218,#22089,#22090);
#18900=AXIS2_PLACEMENT_3D('',#48219,#22091,#22092);
#18901=AXIS2_PLACEMENT_3D('',#48220,#22093,#22094);
#18902=AXIS2_PLACEMENT_3D('',#48221,#22095,#22096);
#18903=AXIS2_PLACEMENT_3D('',#48222,#22097,#22098);
#18904=AXIS2_PLACEMENT_3D('',#48223,#22099,#22100);
#18905=AXIS2_PLACEMENT_3D('',#48224,#22101,#22102);
#18906=AXIS2_PLACEMENT_3D('',#48225,#22103,#22104);
#18907=AXIS2_PLACEMENT_3D('',#48226,#22105,#22106);
#18908=AXIS2_PLACEMENT_3D('',#48227,#22107,#22108);
#18909=AXIS2_PLACEMENT_3D('',#48228,#22109,#22110);
#18910=AXIS2_PLACEMENT_3D('',#48229,#22111,#22112);
#18911=AXIS2_PLACEMENT_3D('',#48230,#22113,#22114);
#18912=AXIS2_PLACEMENT_3D('',#48231,#22115,#22116);
#18913=AXIS2_PLACEMENT_3D('',#48232,#22117,#22118);
#18914=AXIS2_PLACEMENT_3D('',#48233,#22119,#22120);
#18915=AXIS2_PLACEMENT_3D('',#48234,#22121,#22122);
#18916=AXIS2_PLACEMENT_3D('',#48235,#22123,#22124);
#18917=AXIS2_PLACEMENT_3D('',#48236,#22125,#22126);
#18918=AXIS2_PLACEMENT_3D('',#48237,#22127,#22128);
#18919=AXIS2_PLACEMENT_3D('',#48238,#22129,#22130);
#18920=AXIS2_PLACEMENT_3D('',#48239,#22131,#22132);
#18921=AXIS2_PLACEMENT_3D('',#48240,#22133,#22134);
#21841=DIRECTION('axis',(0.,0.,1.));
#21842=DIRECTION('refdir',(1.,0.,0.));
#21843=DIRECTION('center_axis',(0.,1.,0.));
#21844=DIRECTION('ref_axis',(0.,0.,1.));
#21845=DIRECTION('',(0.626301308135395,0.,0.779581087140967));
#21846=DIRECTION('',(-0.488115619572884,0.,0.872778976562211));
#21847=DIRECTION('',(0.571640760429912,0.,0.82050401645276));
#21848=DIRECTION('',(0.987834679513523,0.,-0.155507703829795));
#21849=DIRECTION('',(0.514314959619115,0.,0.857601377279671));
#21850=DIRECTION('',(-0.6024126729918,0.,0.798184797787376));
#21851=DIRECTION('',(0.454591185049047,0.,0.890700204600686));
#21852=DIRECTION('',(0.999808896940505,0.,-0.0195491585141347));
#21853=DIRECTION('',(0.952234407172013,0.,0.305368030084627));
#21854=DIRECTION('center_axis',(0.,1.,0.));
#21855=DIRECTION('ref_axis',(0.,0.,1.));
#21856=DIRECTION('center_axis',(0.,1.,0.));
#21857=DIRECTION('ref_axis',(0.,0.,1.));
#21858=DIRECTION('center_axis',(0.,1.,0.));
#21859=DIRECTION('ref_axis',(0.,0.,1.));
#21860=DIRECTION('',(-0.901654311614274,0.,-0.432457515077943));
#21861=DIRECTION('',(-0.955061656436705,0.,-0.296407207072259));
#21862=DIRECTION('',(-0.364725895711544,0.,0.931114934364932));
#21863=DIRECTION('',(0.678041750029829,0.,0.735023390931532));
#21864=DIRECTION('',(0.957458971062196,0.,-0.288569434854979));
#21865=DIRECTION('center_axis',(0.,1.,0.));
#21866=DIRECTION('ref_axis',(0.,0.,1.));
#21867=DIRECTION('center_axis',(0.,-1.,0.));
#21868=DIRECTION('ref_axis',(0.,0.,-1.));
#21869=DIRECTION('',(0.952234407172013,0.,0.305368030084627));
#21870=DIRECTION('',(0.999808896940505,0.,-0.0195491585141347));
#21871=DIRECTION('',(0.454591185049047,0.,0.890700204600686));
#21872=DIRECTION('',(-0.6024126729918,0.,0.798184797787376));
#21873=DIRECTION('',(0.514314959619115,0.,0.857601377279671));
#21874=DIRECTION('',(0.987834679513523,0.,-0.155507703829795));
#21875=DIRECTION('',(0.571640760429912,0.,0.82050401645276));
#21876=DIRECTION('',(-0.488115619572884,0.,0.872778976562211));
#21877=DIRECTION('',(0.626301308135395,0.,0.779581087140967));
#21878=DIRECTION('',(0.957458971062196,0.,-0.288569434854979));
#21879=DIRECTION('',(0.678041750029829,0.,0.735023390931532));
#21880=DIRECTION('',(-0.364725895711544,0.,0.931114934364932));
#21881=DIRECTION('',(-0.955061656436705,0.,-0.296407207072259));
#21882=DIRECTION('',(-0.901654311614274,0.,-0.432457515077943));
#21883=DIRECTION('center_axis',(0.,-1.,0.));
#21884=DIRECTION('ref_axis',(0.,0.,-1.));
#21885=DIRECTION('center_axis',(0.,-1.,0.));
#21886=DIRECTION('ref_axis',(0.,0.,-1.));
#21887=DIRECTION('center_axis',(0.,-1.,0.));
#21888=DIRECTION('ref_axis',(0.,0.,-1.));
#21889=DIRECTION('center_axis',(0.,-1.,0.));
#21890=DIRECTION('ref_axis',(0.,0.,-1.));
#21891=DIRECTION('center_axis',(-0.155507703829795,0.,-0.987834679513523));
#21892=DIRECTION('ref_axis',(-0.987834679513523,0.,0.155507703829795));
#21893=DIRECTION('',(0.,-1.,0.));
#21894=DIRECTION('',(0.987834679513523,0.,-0.155507703829795));
#21895=DIRECTION('',(0.,-1.,0.));
#21896=DIRECTION('',(0.987834679513523,0.,-0.155507703829795));
#21897=DIRECTION('center_axis',(0.82050401645276,0.,-0.571640760429912));
#21898=DIRECTION('ref_axis',(-0.571640760429912,0.,-0.82050401645276));
#21899=DIRECTION('',(0.,-1.,0.));
#21900=DIRECTION('',(0.571640760429912,0.,0.82050401645276));
#21901=DIRECTION('',(0.571640760429912,0.,0.82050401645276));
#21902=DIRECTION('center_axis',(0.872778976562211,0.,0.488115619572884));
#21903=DIRECTION('ref_axis',(0.488115619572884,0.,-0.872778976562211));
#21904=DIRECTION('',(0.,-1.,0.));
#21905=DIRECTION('',(-0.488115619572884,0.,0.872778976562211));
#21906=DIRECTION('',(-0.488115619572884,0.,0.872778976562211));
#21907=DIRECTION('center_axis',(0.779581087140967,0.,-0.626301308135395));
#21908=DIRECTION('ref_axis',(-0.626301308135395,0.,-0.779581087140967));
#21909=DIRECTION('',(0.,-1.,0.));
#21910=DIRECTION('',(0.626301308135395,0.,0.779581087140967));
#21911=DIRECTION('',(0.626301308135395,0.,0.779581087140967));
#21912=DIRECTION('center_axis',(-0.288569434854979,0.,-0.957458971062195));
#21913=DIRECTION('ref_axis',(-0.957458971062195,0.,0.288569434854979));
#21914=DIRECTION('',(0.,-1.,0.));
#21915=DIRECTION('',(0.957458971062196,0.,-0.288569434854979));
#21916=DIRECTION('',(0.957458971062196,0.,-0.288569434854979));
#21917=DIRECTION('center_axis',(0.735023390931532,0.,-0.678041750029829));
#21918=DIRECTION('ref_axis',(-0.678041750029829,0.,-0.735023390931532));
#21919=DIRECTION('',(0.,-1.,0.));
#21920=DIRECTION('',(0.678041750029829,0.,0.735023390931532));
#21921=DIRECTION('',(0.678041750029829,0.,0.735023390931532));
#21922=DIRECTION('center_axis',(0.931114934364932,0.,0.364725895711544));
#21923=DIRECTION('ref_axis',(0.364725895711544,0.,-0.931114934364932));
#21924=DIRECTION('',(0.,-1.,0.));
#21925=DIRECTION('',(-0.364725895711544,0.,0.931114934364932));
#21926=DIRECTION('',(-0.364725895711544,0.,0.931114934364932));
#21927=DIRECTION('center_axis',(-0.296407207072259,0.,0.955061656436705));
#21928=DIRECTION('ref_axis',(0.955061656436705,0.,0.296407207072259));
#21929=DIRECTION('',(0.,-1.,0.));
#21930=DIRECTION('',(-0.955061656436705,0.,-0.296407207072259));
#21931=DIRECTION('',(-0.955061656436705,0.,-0.296407207072259));
#21932=DIRECTION('center_axis',(-0.432457515077943,0.,0.901654311614274));
#21933=DIRECTION('ref_axis',(0.901654311614274,0.,0.432457515077943));
#21934=DIRECTION('',(0.,1.,0.));
#21935=DIRECTION('',(-0.901654311614274,0.,-0.432457515077943));
#21936=DIRECTION('',(-0.901654311614274,0.,-0.432457515077943));
#21937=DIRECTION('center_axis',(0.,-1.,0.));
#21938=DIRECTION('ref_axis',(-0.96822474174621,0.,0.250081685595898));
#21939=DIRECTION('',(0.,-1.,0.));
#21940=DIRECTION('center_axis',(0.,-1.,0.));
#21941=DIRECTION('ref_axis',(0.,0.,-1.));
#21942=DIRECTION('',(0.,-1.,0.));
#21943=DIRECTION('center_axis',(0.,1.,0.));
#21944=DIRECTION('ref_axis',(0.,0.,1.));
#21945=DIRECTION('center_axis',(0.305368030084627,0.,-0.952234407172013));
#21946=DIRECTION('ref_axis',(-0.952234407172013,0.,-0.305368030084627));
#21947=DIRECTION('',(0.,-1.,0.));
#21948=DIRECTION('',(0.952234407172013,0.,0.305368030084627));
#21949=DIRECTION('',(0.,1.,0.));
#21950=DIRECTION('',(0.952234407172013,0.,0.305368030084627));
#21951=DIRECTION('center_axis',(-0.0195491585141347,0.,-0.999808896940505));
#21952=DIRECTION('ref_axis',(-0.999808896940505,0.,0.0195491585141347));
#21953=DIRECTION('',(0.,-1.,0.));
#21954=DIRECTION('',(0.999808896940505,0.,-0.0195491585141347));
#21955=DIRECTION('',(0.999808896940505,0.,-0.0195491585141347));
#21956=DIRECTION('center_axis',(0.890700204600685,0.,-0.454591185049047));
#21957=DIRECTION('ref_axis',(-0.454591185049047,0.,-0.890700204600686));
#21958=DIRECTION('',(0.,-1.,0.));
#21959=DIRECTION('',(0.454591185049047,0.,0.890700204600686));
#21960=DIRECTION('',(0.454591185049047,0.,0.890700204600686));
#21961=DIRECTION('center_axis',(0.798184797787376,0.,0.6024126729918));
#21962=DIRECTION('ref_axis',(0.6024126729918,0.,-0.798184797787376));
#21963=DIRECTION('',(0.,-1.,0.));
#21964=DIRECTION('',(-0.6024126729918,0.,0.798184797787376));
#21965=DIRECTION('',(-0.6024126729918,0.,0.798184797787376));
#21966=DIRECTION('center_axis',(0.857601377279671,0.,-0.514314959619115));
#21967=DIRECTION('ref_axis',(-0.514314959619115,0.,-0.857601377279671));
#21968=DIRECTION('',(0.514314959619115,0.,0.857601377279671));
#21969=DIRECTION('',(0.514314959619115,0.,0.857601377279671));
#21970=DIRECTION('center_axis',(0.,-1.,0.));
#21971=DIRECTION('ref_axis',(0.,0.,-1.));
#21972=DIRECTION('center_axis',(0.,1.,0.));
#21973=DIRECTION('ref_axis',(0.,0.,1.));
#21974=DIRECTION('center_axis',(0.,1.,0.));
#21975=DIRECTION('ref_axis',(0.,0.,1.));
#21976=DIRECTION('',(0.,-1.,0.));
#21977=DIRECTION('center_axis',(0.,-1.,0.));
#21978=DIRECTION('ref_axis',(0.,0.,-1.));
#21979=DIRECTION('center_axis',(-0.488115619572884,0.,0.872778976562211));
#21980=DIRECTION('ref_axis',(0.872778976562211,0.,0.488115619572884));
#21981=DIRECTION('center_axis',(0.0492674350094236,0.,0.998785622567522));
#21982=DIRECTION('ref_axis',(-0.998785622567522,0.,0.0492674350094236));
#21983=DIRECTION('center_axis',(0.0833383631889745,0.,0.996521307961341));
#21984=DIRECTION('ref_axis',(-0.996521307961341,0.,0.0833383631889746));
#21985=DIRECTION('center_axis',(0.626301308135395,0.,0.779581087140967));
#21986=DIRECTION('ref_axis',(0.779581087140968,0.,-0.626301308135395));
#21987=DIRECTION('center_axis',(0.955149485630946,0.,0.29612406200601));
#21988=DIRECTION('ref_axis',(-0.29612406200601,0.,0.955149485630946));
#21989=DIRECTION('center_axis',(0.626301308135395,0.,0.779581087140967));
#21990=DIRECTION('ref_axis',(0.779581087140968,0.,-0.626301308135395));
#21991=DIRECTION('center_axis',(0.955149485630946,0.,0.29612406200601));
#21992=DIRECTION('ref_axis',(0.29612406200601,0.,-0.955149485630946));
#21993=DIRECTION('center_axis',(0.0833383631889745,0.,0.996521307961341));
#21994=DIRECTION('ref_axis',(0.996521307961341,0.,-0.0833383631889746));
#21995=DIRECTION('center_axis',(-0.488115619572884,0.,0.872778976562211));
#21996=DIRECTION('ref_axis',(0.872778976562211,0.,0.488115619572884));
#21997=DIRECTION('center_axis',(0.0492674350094236,0.,0.998785622567522));
#21998=DIRECTION('ref_axis',(0.998785622567522,0.,-0.0492674350094236));
#21999=DIRECTION('center_axis',(0.571640760429912,0.,0.82050401645276));
#22000=DIRECTION('ref_axis',(0.82050401645276,0.,-0.571640760429912));
#22001=DIRECTION('center_axis',(0.919859028046646,0.,0.392249115385974));
#22002=DIRECTION('ref_axis',(-0.392249115385974,0.,0.919859028046646));
#22003=DIRECTION('center_axis',(0.957458971062196,0.,-0.288569434854979));
#22004=DIRECTION('ref_axis',(-0.288569434854979,0.,-0.957458971062195));
#22005=DIRECTION('center_axis',(0.964702659073528,0.,0.263341564468019));
#22006=DIRECTION('ref_axis',(-0.263341564468019,0.,0.964702659073528));
#22007=DIRECTION('center_axis',(0.957458971062196,0.,-0.288569434854979));
#22008=DIRECTION('ref_axis',(-0.288569434854979,0.,-0.957458971062195));
#22009=DIRECTION('center_axis',(0.964702659073528,0.,0.263341564468019));
#22010=DIRECTION('ref_axis',(0.263341564468019,0.,-0.964702659073528));
#22011=DIRECTION('center_axis',(0.571640760429912,0.,0.82050401645276));
#22012=DIRECTION('ref_axis',(0.82050401645276,0.,-0.571640760429912));
#22013=DIRECTION('center_axis',(0.919859028046646,0.,0.392249115385974));
#22014=DIRECTION('ref_axis',(0.392249115385974,0.,-0.919859028046646));
#22015=DIRECTION('center_axis',(0.987834679513523,0.,-0.155507703829795));
#22016=DIRECTION('ref_axis',(-0.155507703829795,0.,-0.987834679513523));
#22017=DIRECTION('center_axis',(0.905930950538282,0.,0.423425451356913));
#22018=DIRECTION('ref_axis',(0.423425451356913,0.,-0.905930950538282));
#22019=DIRECTION('center_axis',(0.678041750029829,0.,0.735023390931532));
#22020=DIRECTION('ref_axis',(0.735023390931532,0.,-0.678041750029829));
#22021=DIRECTION('center_axis',(0.184809846851629,0.,0.982774297845989));
#22022=DIRECTION('ref_axis',(-0.982774297845989,0.,0.184809846851629));
#22023=DIRECTION('center_axis',(0.678041750029829,0.,0.735023390931532));
#22024=DIRECTION('ref_axis',(0.735023390931532,0.,-0.678041750029829));
#22025=DIRECTION('center_axis',(0.184809846851629,0.,0.982774297845989));
#22026=DIRECTION('ref_axis',(0.982774297845989,0.,-0.184809846851629));
#22027=DIRECTION('center_axis',(0.987834679513523,0.,-0.155507703829795));
#22028=DIRECTION('ref_axis',(-0.155507703829795,0.,-0.987834679513523));
#22029=DIRECTION('center_axis',(0.905930950538282,0.,0.423425451356913));
#22030=DIRECTION('ref_axis',(0.423425451356913,0.,-0.905930950538282));
#22031=DIRECTION('center_axis',(0.514314959619115,0.,0.857601377279671));
#22032=DIRECTION('ref_axis',(0.857601377279671,0.,-0.514314959619115));
#22033=DIRECTION('center_axis',(-0.0531308220811139,0.,0.998587560379652));
#22034=DIRECTION('ref_axis',(-0.998587560379652,0.,-0.0531308220811139));
#22035=DIRECTION('center_axis',(-0.364725895711544,0.,0.931114934364932));
#22036=DIRECTION('ref_axis',(0.931114934364932,0.,0.364725895711544));
#22037=DIRECTION('center_axis',(-0.90120055904943,0.,0.433402298527587));
#22038=DIRECTION('ref_axis',(-0.433402298527587,0.,-0.90120055904943));
#22039=DIRECTION('center_axis',(-0.364725895711544,0.,0.931114934364932));
#22040=DIRECTION('ref_axis',(0.931114934364932,0.,0.364725895711544));
#22041=DIRECTION('center_axis',(-0.90120055904943,0.,0.433402298527587));
#22042=DIRECTION('ref_axis',(0.433402298527587,0.,0.90120055904943));
#22043=DIRECTION('center_axis',(0.514314959619115,0.,0.857601377279671));
#22044=DIRECTION('ref_axis',(0.857601377279671,0.,-0.514314959619115));
#22045=DIRECTION('center_axis',(-0.0531308220811139,0.,0.998587560379652));
#22046=DIRECTION('ref_axis',(-0.998587560379652,0.,-0.0531308220811139));
#22047=DIRECTION('center_axis',(-0.6024126729918,0.,0.798184797787376));
#22048=DIRECTION('ref_axis',(0.798184797787376,0.,0.6024126729918));
#22049=DIRECTION('center_axis',(-0.087192735929436,0.,0.996191460915591));
#22050=DIRECTION('ref_axis',(-0.996191460915591,0.,-0.087192735929436));
#22051=DIRECTION('center_axis',(-0.955061656436705,0.,-0.296407207072259));
#22052=DIRECTION('ref_axis',(-0.296407207072259,0.,0.955061656436705));
#22053=DIRECTION('center_axis',(-0.930846909046263,0.,-0.365409403161739));
#22054=DIRECTION('ref_axis',(0.365409403161739,0.,-0.930846909046263));
#22055=DIRECTION('center_axis',(-0.955061656436705,0.,-0.296407207072259));
#22056=DIRECTION('ref_axis',(-0.296407207072259,0.,0.955061656436705));
#22057=DIRECTION('center_axis',(-0.930846909046263,0.,-0.365409403161739));
#22058=DIRECTION('ref_axis',(-0.365409403161739,0.,0.930846909046263));
#22059=DIRECTION('center_axis',(-0.6024126729918,0.,0.798184797787376));
#22060=DIRECTION('ref_axis',(0.798184797787376,0.,0.6024126729918));
#22061=DIRECTION('center_axis',(-0.087192735929436,0.,0.996191460915591));
#22062=DIRECTION('ref_axis',(0.996191460915591,0.,0.087192735929436));
#22063=DIRECTION('center_axis',(0.454591185049047,0.,0.890700204600686));
#22064=DIRECTION('ref_axis',(0.890700204600686,0.,-0.454591185049047));
#22065=DIRECTION('center_axis',(0.857880163767375,0.,0.513849807448113));
#22066=DIRECTION('ref_axis',(-0.513849807448113,0.,0.857880163767375));
#22067=DIRECTION('center_axis',(-0.901654311614274,0.,-0.432457515077943));
#22068=DIRECTION('ref_axis',(-0.432457515077943,0.,0.901654311614274));
#22069=DIRECTION('center_axis',(-0.901654311614274,0.,-0.432457515077943));
#22070=DIRECTION('ref_axis',(-0.432457515077943,0.,0.901654311614274));
#22071=DIRECTION('center_axis',(0.,-1.,0.));
#22072=DIRECTION('ref_axis',(0.,0.,-1.));
#22073=DIRECTION('center_axis',(0.,-1.,0.));
#22074=DIRECTION('ref_axis',(0.,0.,-1.));
#22075=DIRECTION('center_axis',(0.,1.,0.));
#22076=DIRECTION('ref_axis',(0.,0.,1.));
#22077=DIRECTION('center_axis',(-0.901654311614274,0.,-0.432457515077943));
#22078=DIRECTION('ref_axis',(-0.432457515077943,0.,0.901654311614274));
#22079=DIRECTION('center_axis',(-0.901654311614274,0.,-0.432457515077943));
#22080=DIRECTION('ref_axis',(-0.432457515077943,0.,0.901654311614274));
#22081=DIRECTION('center_axis',(0.454591185049047,0.,0.890700204600686));
#22082=DIRECTION('ref_axis',(0.890700204600686,0.,-0.454591185049047));
#22083=DIRECTION('center_axis',(0.857880163767375,0.,0.513849807448113));
#22084=DIRECTION('ref_axis',(0.513849807448113,0.,-0.857880163767375));
#22085=DIRECTION('center_axis',(0.999808896940505,0.,-0.0195491585141347));
#22086=DIRECTION('ref_axis',(-0.0195491585141347,0.,-0.999808896940505));
#22087=DIRECTION('center_axis',(0.989449877530115,0.,0.144875601312438));
#22088=DIRECTION('ref_axis',(-0.144875601312438,0.,0.989449877530115));
#22089=DIRECTION('center_axis',(0.,1.,0.));
#22090=DIRECTION('ref_axis',(-0.302115636055689,0.,-0.95327128481386));
#22091=DIRECTION('center_axis',(0.48796543950748,0.,-0.872862950208262));
#22092=DIRECTION('ref_axis',(-0.872862950208263,0.,-0.48796543950748));
#22093=DIRECTION('center_axis',(0.,-1.,0.));
#22094=DIRECTION('ref_axis',(0.,0.,-1.));
#22095=DIRECTION('center_axis',(0.487965439507477,3.78543962759162E-15,
-0.872862950208264));
#22096=DIRECTION('ref_axis',(-0.872862950208264,-3.40301281036919E-32,-0.487965439507477));
#22097=DIRECTION('center_axis',(0.999808896940505,0.,-0.0195491585141347));
#22098=DIRECTION('ref_axis',(-0.0195491585141347,0.,-0.999808896940505));
#22099=DIRECTION('center_axis',(0.989449877530115,0.,0.144875601312438));
#22100=DIRECTION('ref_axis',(0.144875601312438,0.,-0.989449877530115));
#22101=DIRECTION('center_axis',(0.952234407172013,0.,0.305368030084627));
#22102=DIRECTION('ref_axis',(0.305368030084627,0.,-0.952234407172013));
#22103=DIRECTION('center_axis',(-0.952234407172012,0.,-0.30536803008463));
#22104=DIRECTION('ref_axis',(-0.30536803008463,0.,0.952234407172012));
#22105=DIRECTION('center_axis',(0.,1.,0.));
#22106=DIRECTION('ref_axis',(-0.96822474174621,0.,0.250081685595898));
#22107=DIRECTION('center_axis',(0.849631715069657,0.,0.527376477241631));
#22108=DIRECTION('ref_axis',(0.527376477241631,0.,-0.849631715069657));
#22109=DIRECTION('center_axis',(0.,-1.,0.));
#22110=DIRECTION('ref_axis',(-0.96822474174621,0.,0.250081685595898));
#22111=DIRECTION('center_axis',(0.849631715069657,0.,0.527376477241631));
#22112=DIRECTION('ref_axis',(0.527376477241631,0.,-0.849631715069657));
#22113=DIRECTION('center_axis',(0.952234407172013,0.,0.305368030084627));
#22114=DIRECTION('ref_axis',(0.305368030084627,0.,-0.952234407172013));
#22115=DIRECTION('center_axis',(-0.952234407172012,1.3243227265015E-15,
-0.30536803008463));
#22116=DIRECTION('ref_axis',(-0.30536803008463,4.13937419839926E-32,0.952234407172012));
#22117=DIRECTION('center_axis',(0.,1.,0.));
#22118=DIRECTION('ref_axis',(0.,0.,1.));
#22119=DIRECTION('center_axis',(0.,1.,0.));
#22120=DIRECTION('ref_axis',(0.,0.,1.));
#22121=DIRECTION('center_axis',(0.,-1.,0.));
#22122=DIRECTION('ref_axis',(0.,0.,-1.));
#22123=DIRECTION('center_axis',(0.,-1.,0.));
#22124=DIRECTION('ref_axis',(0.,0.,-1.));
#22125=DIRECTION('center_axis',(0.,-1.,0.));
#22126=DIRECTION('ref_axis',(0.,0.,-1.));
#22127=DIRECTION('center_axis',(0.,-1.,0.));
#22128=DIRECTION('ref_axis',(0.,0.,-1.));
#22129=DIRECTION('center_axis',(-1.,0.,0.));
#22130=DIRECTION('ref_axis',(0.,0.,1.));
#22131=DIRECTION('center_axis',(0.,1.,0.));
#22132=DIRECTION('ref_axis',(0.,0.,1.));
#22133=DIRECTION('center_axis',(-1.,0.,0.));
#22134=DIRECTION('ref_axis',(0.,0.,-1.));
#47984=CARTESIAN_POINT('',(0.,0.,0.));
#47985=CARTESIAN_POINT('Origin',(0.00625,0.013,-2.29621274840129E-18));
#47986=CARTESIAN_POINT('',(0.00310513229246118,0.013,0.00782534372202691));
#47987=CARTESIAN_POINT('',(0.00283397885998211,0.013,0.00748782871937848));
#47988=CARTESIAN_POINT('',(0.000517972272646041,0.013,0.00460500712899027));
#47989=CARTESIAN_POINT('',(0.00343760106241995,0.013,0.00640851728792926));
#47990=CARTESIAN_POINT('',(0.00683781203254235,0.013,0.000328743292588178));
#47991=CARTESIAN_POINT('',(0.00334867942190192,0.013,0.00628088369661617));
#47992=CARTESIAN_POINT('',(0.00135080799850545,0.013,0.00341324086789248));
#47993=CARTESIAN_POINT('',(0.00212708576461598,0.013,0.00647319039387763));
#47994=CARTESIAN_POINT('',(0.00714468201094909,0.013,0.00568330633008214));
#47995=CARTESIAN_POINT('',(0.00190441615676979,0.013,0.00610189696988579));
#47996=CARTESIAN_POINT('',(0.00036250172514288,0.013,0.00353081107110126));
#47997=CARTESIAN_POINT('',(0.00264938241039218,0.013,0.00511483151597876));
#47998=CARTESIAN_POINT('',(0.00641544862510175,0.013,0.000124868763181971));
#47999=CARTESIAN_POINT('',(0.00257866842927369,0.013,0.00497627854900125));
#48000=CARTESIAN_POINT('',(0.00132244326030609,0.013,0.0025149021479097));
#48001=CARTESIAN_POINT('',(0.00139305626828131,0.013,0.00499946069925261));
#48002=CARTESIAN_POINT('',(0.00634586039595321,0.013,0.00490261903953383));
#48003=CARTESIAN_POINT('',(-0.00848709681638249,0.013,0.00183103613732295));
#48004=CARTESIAN_POINT('',(0.00434333886907659,0.013,0.00594557436539644));
#48005=CARTESIAN_POINT('',(-0.00853149850581388,0.013,0.00181051559890248));
#48006=CARTESIAN_POINT('Origin',(-0.00842602321036556,0.013,0.00164058925588855));
#48007=CARTESIAN_POINT('',(-0.00804781744366059,0.013,0.00368315161531047));
#48008=CARTESIAN_POINT('Origin',(-0.00926982557395217,0.013,0.003));
#48009=CARTESIAN_POINT('',(-0.00778675335060335,0.013,0.00360041384088911));
#48010=CARTESIAN_POINT('Origin',(-0.00787324485361894,0.013,0.00378074470321196));
#48011=CARTESIAN_POINT('',(4.52079337442143E-5,0.013,0.00735683187337399));
#48012=CARTESIAN_POINT('',(0.00222095414696891,0.013,0.00840037792943047));
#48013=CARTESIAN_POINT('',(0.00400212262074066,0.013,0.00858487618139458));
#48014=CARTESIAN_POINT('',(0.0036222395132741,0.013,0.00846697793876363));
#48015=CARTESIAN_POINT('',(0.00439463505993757,0.013,0.00758282450818601));
#48016=CARTESIAN_POINT('',(0.00721658525161907,0.013,0.000378619930437244));
#48017=CARTESIAN_POINT('',(0.00428916220193663,0.013,0.00746848786485147));
#48018=CARTESIAN_POINT('',(0.00146851978854034,0.013,0.00441080277214348));
#48019=CARTESIAN_POINT('',(0.00815021035144082,0.013,0.00630480303226358));
#48020=CARTESIAN_POINT('',(-0.00926982557395217,0.013,0.0024));
#48021=CARTESIAN_POINT('Origin',(-0.00926982557395217,0.013,0.003));
#48022=CARTESIAN_POINT('Origin',(-0.00926982557395217,0.001,0.003));
#48023=CARTESIAN_POINT('',(-0.00848709681638249,0.001,0.00183103613732295));
#48024=CARTESIAN_POINT('',(0.00139305626828131,0.001,0.00499946069925261));
#48025=CARTESIAN_POINT('',(-0.00885692281820857,0.001,0.001712438198831));
#48026=CARTESIAN_POINT('',(0.00257866842927369,0.001,0.00497627854900125));
#48027=CARTESIAN_POINT('',(-0.00922667024031924,0.001,0.0052071070980081));
#48028=CARTESIAN_POINT('',(0.00264938241039218,0.001,0.00511483151597876));
#48029=CARTESIAN_POINT('',(-0.000670064127940984,0.001,-0.00138910390576812));
#48030=CARTESIAN_POINT('',(0.00190441615676979,0.001,0.00610189696988579));
#48031=CARTESIAN_POINT('',(-0.000659221951814677,0.001,0.00949866642219173));
#48032=CARTESIAN_POINT('',(0.00212708576461598,0.001,0.00647319039387763));
#48033=CARTESIAN_POINT('',(-0.00241956898424355,0.001,-0.00110819004569721));
#48034=CARTESIAN_POINT('',(0.00334867942190192,0.001,0.00628088369661617));
#48035=CARTESIAN_POINT('',(-0.00846068082425976,0.001,0.0081399462843802));
#48036=CARTESIAN_POINT('',(0.00343760106241995,0.001,0.00640851728792926));
#48037=CARTESIAN_POINT('',(-0.0023135538114868,0.001,-0.00184639733665676));
#48038=CARTESIAN_POINT('',(0.00283397885998211,0.001,0.00748782871937848));
#48039=CARTESIAN_POINT('',(0.00186205600079768,0.001,0.00922568303979271));
#48040=CARTESIAN_POINT('',(0.00310513229246119,0.001,0.00782534372202692));
#48041=CARTESIAN_POINT('',(-0.0041049730035732,0.001,-0.00114934889328565));
#48042=CARTESIAN_POINT('',(0.00428916220193663,0.001,0.00746848786485147));
#48043=CARTESIAN_POINT('',(-0.0069061235431728,0.001,0.0108426452733117));
#48044=CARTESIAN_POINT('',(0.00439463505993757,0.001,0.00758282450818601));
#48045=CARTESIAN_POINT('',(-0.00417144472326108,0.001,-0.00170313614093291));
#48046=CARTESIAN_POINT('',(0.00400212262074066,0.001,0.00858487618139458));
#48047=CARTESIAN_POINT('',(0.00413325559518032,0.001,0.00825010458353409));
#48048=CARTESIAN_POINT('',(4.52079337442122E-5,0.001,0.00735683187337399));
#48049=CARTESIAN_POINT('',(-0.00968479566385333,0.001,0.00433708631901139));
#48050=CARTESIAN_POINT('',(-0.00778675335060335,0.001,0.00360041384088911));
#48051=CARTESIAN_POINT('',(-0.00922657982244437,0.001,0.00290983456883857));
#48052=CARTESIAN_POINT('',(-0.00804781744366059,0.001,0.00368315161531047));
#48053=CARTESIAN_POINT('Origin',(-0.00787324485361894,0.001,0.00378074470321196));
#48054=CARTESIAN_POINT('',(-0.00853149850581388,0.001,0.00181051559890248));
#48055=CARTESIAN_POINT('Origin',(-0.00926982557395217,0.001,0.003));
#48056=CARTESIAN_POINT('Origin',(-0.00842602321036556,0.001,0.00164058925588855));
#48057=CARTESIAN_POINT('',(-0.00926982557395217,0.001,0.0036));
#48058=CARTESIAN_POINT('Origin',(-0.00926982557395217,0.001,0.003));
#48059=CARTESIAN_POINT('Origin',(0.00217815846891078,0.0298951219150416,
0.00636391887181847));
#48060=CARTESIAN_POINT('',(0.00339495317277858,0.0129,0.00617236763925401));
#48061=CARTESIAN_POINT('',(0.00339495317277858,0.0011,0.00617236763925401));
#48062=CARTESIAN_POINT('',(0.00339495317277858,0.0298951219150416,0.00617236763925401));
#48063=CARTESIAN_POINT('',(0.00217815846891078,0.0011,0.00636391887181847));
#48064=CARTESIAN_POINT('',(0.00217815846891078,0.0011,0.00636391887181847));
#48065=CARTESIAN_POINT('',(0.00217815846891078,0.0129,0.00636391887181847));
#48066=CARTESIAN_POINT('',(0.00217815846891078,0.0298951219150416,0.00636391887181847));
#48067=CARTESIAN_POINT('',(0.00217815846891078,0.0129,0.00636391887181847));
#48068=CARTESIAN_POINT('Origin',(0.00339495317277858,0.0298951219150416,
0.00617236763925401));
#48069=CARTESIAN_POINT('',(0.00355542811483384,0.0129,0.00640270519320544));
#48070=CARTESIAN_POINT('',(0.00355542811483384,0.0011,0.00640270519320544));
#48071=CARTESIAN_POINT('',(0.00355542811483384,0.0298951219150416,0.00640270519320544));
#48072=CARTESIAN_POINT('',(0.00339495317277858,0.0011,0.00617236763925401));
#48073=CARTESIAN_POINT('',(0.00339495317277858,0.0129,0.00617236763925401));
#48074=CARTESIAN_POINT('Origin',(0.00355542811483384,0.0298951219150416,
0.00640270519320544));
#48075=CARTESIAN_POINT('',(0.00295417720403981,0.0129,0.00747777661796151));
#48076=CARTESIAN_POINT('',(0.00295417720403981,0.0011,0.00747777661796151));
#48077=CARTESIAN_POINT('',(0.00295417720403981,0.0298951219150416,0.00747777661796151));
#48078=CARTESIAN_POINT('',(0.00355542811483384,0.0011,0.00640270519320544));
#48079=CARTESIAN_POINT('',(0.00355542811483384,0.0129,0.00640270519320544));
#48080=CARTESIAN_POINT('Origin',(0.00295417720403981,0.0298951219150416,
0.00747777661796151));
#48081=CARTESIAN_POINT('',(0.00314085016583167,0.0129,0.0077101355618168));
#48082=CARTESIAN_POINT('',(0.00314085016583167,0.0011,0.0077101355618168));
#48083=CARTESIAN_POINT('',(0.00314085016583167,0.0298951219150416,0.0077101355618168));
#48084=CARTESIAN_POINT('',(0.00295417720403981,0.0011,0.00747777661796151));
#48085=CARTESIAN_POINT('',(0.00295417720403981,0.0129,0.00747777661796151));
#48086=CARTESIAN_POINT('Origin',(0.00314085016583167,0.0298951219150416,
0.0077101355618168));
#48087=CARTESIAN_POINT('',(0.00432022868869639,0.0129,0.00735468159030551));
#48088=CARTESIAN_POINT('',(0.00432022868869639,0.0011,0.00735468159030551));
#48089=CARTESIAN_POINT('',(0.00432022868869639,0.0298951219150416,0.00735468159030551));
#48090=CARTESIAN_POINT('',(0.00314085016583167,0.0011,0.0077101355618168));
#48091=CARTESIAN_POINT('',(0.00314085016583167,0.0129,0.0077101355618168));
#48092=CARTESIAN_POINT('Origin',(0.00432022868869639,0.0298951219150416,
0.00735468159030551));
#48093=CARTESIAN_POINT('',(0.00451057325136412,0.0129,0.007561022432726));
#48094=CARTESIAN_POINT('',(0.00451057325136412,0.0011,0.007561022432726));
#48095=CARTESIAN_POINT('',(0.00451057325136412,0.0298951219150416,0.007561022432726));
#48096=CARTESIAN_POINT('',(0.00432022868869639,0.0011,0.00735468159030551));
#48097=CARTESIAN_POINT('',(0.00432022868869639,0.0129,0.00735468159030551));
#48098=CARTESIAN_POINT('Origin',(0.00451057325136412,0.0298951219150416,
0.007561022432726));
#48099=CARTESIAN_POINT('',(0.0040613112974471,0.0129,0.00870795090600599));
#48100=CARTESIAN_POINT('',(0.0040613112974471,0.0011,0.00870795090600599));
#48101=CARTESIAN_POINT('',(0.0040613112974471,0.0298951219150416,0.00870795090600599));
#48102=CARTESIAN_POINT('',(0.00451057325136412,0.0011,0.007561022432726));
#48103=CARTESIAN_POINT('',(0.00451057325136412,0.0129,0.007561022432726));
#48104=CARTESIAN_POINT('Origin',(0.0040613112974471,0.0298951219150416,
0.00870795090600599));
#48105=CARTESIAN_POINT('',(8.56902727468245E-6,0.0129,0.00745016612406076));
#48106=CARTESIAN_POINT('',(8.56902727468245E-6,0.0011,0.00745016612406076));
#48107=CARTESIAN_POINT('',(8.56902727468245E-6,0.0298951219150416,0.00745016612406076));
#48108=CARTESIAN_POINT('',(0.0040613112974471,0.0011,0.00870795090600599));
#48109=CARTESIAN_POINT('',(0.0040613112974471,0.0129,0.00870795090600599));
#48110=CARTESIAN_POINT('Origin',(8.56902727468245E-6,0.0298951219150416,
0.00745016612406076));
#48111=CARTESIAN_POINT('',(-0.00782999910211115,0.0129,0.00369057927205054));
#48112=CARTESIAN_POINT('',(-0.00782999910211115,0.0011,0.00369057927205054));
#48113=CARTESIAN_POINT('',(-0.00782999910211115,0.001,0.00369057927205053));
#48114=CARTESIAN_POINT('',(8.56902727468245E-6,0.0011,0.00745016612406076));
#48115=CARTESIAN_POINT('',(8.56902727468245E-6,0.0129,0.00745016612406076));
#48116=CARTESIAN_POINT('Origin',(-0.00926982557395217,0.0298951219150416,
0.003));
#48117=CARTESIAN_POINT('',(-0.00847876085808972,0.0129,0.00172555242739552));
#48118=CARTESIAN_POINT('',(-0.00847876085808972,0.0011,0.00172555242739552));
#48119=CARTESIAN_POINT('',(-0.00847876085808972,0.0298951219150416,0.00172555242739552));
#48120=CARTESIAN_POINT('',(-0.00796053114863977,0.0011,0.00373194815926121));
#48121=CARTESIAN_POINT('Origin',(-0.00926982557395217,0.0011,0.003));
#48122=CARTESIAN_POINT('',(-0.00796053114863977,0.0129,0.00373194815926121));
#48123=CARTESIAN_POINT('',(-0.00796053114863977,0.0298951219150416,0.00373194815926121));
#48124=CARTESIAN_POINT('Origin',(-0.00926982557395217,0.0129,0.003));
#48125=CARTESIAN_POINT('Origin',(-0.00846848477354713,0.0298951219150416,
0.00173198859563243));
#48126=CARTESIAN_POINT('',(0.0014077431500399,0.0129,0.00489915441423508));
#48127=CARTESIAN_POINT('',(0.0014077431500399,0.0011,0.00489915441423508));
#48128=CARTESIAN_POINT('',(0.0014077431500399,0.0298951219150416,0.00489915441423508));
#48129=CARTESIAN_POINT('',(-0.00845656001337402,0.0011,0.00173581269660575));
#48130=CARTESIAN_POINT('',(-0.00846848477354713,0.0011,0.00173198859563243));
#48131=CARTESIAN_POINT('',(-0.00845656001337402,0.0129,0.00173581269660575));
#48132=CARTESIAN_POINT('',(-0.00845656001337402,0.013,0.00173581269660575));
#48133=CARTESIAN_POINT('',(-0.00846848477354713,0.0129,0.00173198859563243));
#48134=CARTESIAN_POINT('Origin',(0.0014077431500399,0.0298951219150416,
0.00489915441423508));
#48135=CARTESIAN_POINT('',(0.00263928745184173,0.0129,0.00487507415765127));
#48136=CARTESIAN_POINT('',(0.00263928745184173,0.0011,0.00487507415765127));
#48137=CARTESIAN_POINT('',(0.00263928745184173,0.0298951219150416,0.00487507415765127));
#48138=CARTESIAN_POINT('',(0.0014077431500399,0.0011,0.00489915441423508));
#48139=CARTESIAN_POINT('',(0.0014077431500399,0.0129,0.00489915441423508));
#48140=CARTESIAN_POINT('Origin',(0.00263928745184173,0.0298951219150416,
0.00487507415765127));
#48141=CARTESIAN_POINT('',(0.00276690342874427,0.0129,0.00512511767031892));
#48142=CARTESIAN_POINT('',(0.00276690342874427,0.0011,0.00512511767031892));
#48143=CARTESIAN_POINT('',(0.00276690342874427,0.0298951219150416,0.00512511767031892));
#48144=CARTESIAN_POINT('',(0.00263928745184173,0.0011,0.00487507415765127));
#48145=CARTESIAN_POINT('',(0.00263928745184173,0.0129,0.00487507415765127));
#48146=CARTESIAN_POINT('Origin',(0.00276690342874427,0.0298951219150416,
0.00512511767031892));
#48147=CARTESIAN_POINT('',(0.00202486372793092,0.0129,0.00610830550002113));
#48148=CARTESIAN_POINT('',(0.00202486372793092,0.0011,0.00610830550002113));
#48149=CARTESIAN_POINT('',(0.00202486372793092,0.0298951219150416,0.00610830550002113));
#48150=CARTESIAN_POINT('',(0.00276690342874427,0.0011,0.00512511767031892));
#48151=CARTESIAN_POINT('',(0.00276690342874427,0.0129,0.00512511767031892));
#48152=CARTESIAN_POINT('Origin',(0.00202486372793092,0.0298951219150416,
0.00610830550002113));
#48153=CARTESIAN_POINT('',(0.00202486372793092,0.0011,0.00610830550002113));
#48154=CARTESIAN_POINT('',(0.00202486372793092,0.0129,0.00610830550002113));
#48155=CARTESIAN_POINT('Origin',(-0.00926982557395217,0.0172006855706717,
0.003));
#48156=CARTESIAN_POINT('',(-0.00926982557395217,0.0129,0.0035));
#48157=CARTESIAN_POINT('',(-0.00926982557395217,0.0129,0.0025));
#48158=CARTESIAN_POINT('Origin',(-0.00926982557395217,0.0129,0.003));
#48159=CARTESIAN_POINT('Origin',(-0.00926982557395217,0.0129,0.003));
#48160=CARTESIAN_POINT('',(-0.00926982557395217,0.0011,0.0035));
#48161=CARTESIAN_POINT('',(-0.00926982557395217,0.0172006855706717,0.0035));
#48162=CARTESIAN_POINT('Origin',(-0.00926982557395217,0.0011,0.003));
#48163=CARTESIAN_POINT('Origin',(0.00346815021717762,0.0129,0.00635389363124816));
#48164=CARTESIAN_POINT('Origin',(0.00343760106241995,0.0129,0.00640851728792926));
#48165=CARTESIAN_POINT('Origin',(0.00283397885998211,0.0129,0.00748782871937848));
#48166=CARTESIAN_POINT('Origin',(0.00287621909532571,0.0129,0.00754040674877505));
#48167=CARTESIAN_POINT('Origin',(0.00310513229246118,0.0129,0.00782534372202691));
#48168=CARTESIAN_POINT('Origin',(-0.0041049730035732,0.0011,-0.00114934889328566));
#48169=CARTESIAN_POINT('Origin',(0.00310513229246118,0.0011,0.00782534372202692));
#48170=CARTESIAN_POINT('Origin',(0.00283397885998211,0.0011,0.00748782871937847));
#48171=CARTESIAN_POINT('Origin',(0.00186205600079768,0.0011,0.00922568303979271));
#48172=CARTESIAN_POINT('Origin',(0.00343760106241995,0.0011,0.00640851728792926));
#48173=CARTESIAN_POINT('Origin',(0.00331290277113331,0.0129,0.006229531715297));
#48174=CARTESIAN_POINT('Origin',(0.00334867942190192,0.0129,0.00628088369661617));
#48175=CARTESIAN_POINT('Origin',(0.00316970710931718,0.0129,0.00780588145892302));
#48176=CARTESIAN_POINT('Origin',(0.00428916220193663,0.0129,0.00746848786485147));
#48177=CARTESIAN_POINT('Origin',(-0.0069061235431728,0.0011,0.0108426452733117));
#48178=CARTESIAN_POINT('Origin',(0.00428916220193663,0.0011,0.00746848786485147));
#48179=CARTESIAN_POINT('Origin',(-0.0023135538114868,0.0011,-0.00184639733665676));
#48180=CARTESIAN_POINT('Origin',(0.00334867942190192,0.0011,0.00628088369661617));
#48181=CARTESIAN_POINT('Origin',(0.00219370923929376,0.0129,0.00646270233976982));
#48182=CARTESIAN_POINT('Origin',(0.00212708576461598,0.0129,0.00647319039387763));
#48183=CARTESIAN_POINT('Origin',(0.00424672634960323,0.0129,0.00742248576530849));
#48184=CARTESIAN_POINT('Origin',(0.00439463505993757,0.0129,0.00758282450818601));
#48185=CARTESIAN_POINT('Origin',(-0.00417144472326108,0.0011,-0.00170313614093291));
#48186=CARTESIAN_POINT('Origin',(0.00439463505993757,0.0011,0.00758282450818601));
#48187=CARTESIAN_POINT('Origin',(-0.00846068082425976,0.0011,0.0081399462843802));
#48188=CARTESIAN_POINT('Origin',(0.00212708576461597,0.0011,0.00647319039387763));
#48189=CARTESIAN_POINT('Origin',(0.00193910359020296,0.0129,0.00615973699598304));
#48190=CARTESIAN_POINT('Origin',(0.00190441615676979,0.0129,0.00610189696988579));
#48191=CARTESIAN_POINT('Origin',(0.00441746175792763,0.0129,0.00752454984315485));
#48192=CARTESIAN_POINT('Origin',(0.00400212262074066,0.0129,0.00858487618139458));
#48193=CARTESIAN_POINT('Origin',(0.00413325559518032,0.0011,0.00825010458353409));
#48194=CARTESIAN_POINT('Origin',(0.00400212262074067,0.0011,0.00858487618139459));
#48195=CARTESIAN_POINT('Origin',(-0.00241956898424355,0.0011,-0.00110819004569721));
#48196=CARTESIAN_POINT('Origin',(0.00190441615676979,0.0011,0.00610189696988579));
#48197=CARTESIAN_POINT('Origin',(0.00268708494896553,0.0129,0.00506487640301974));
#48198=CARTESIAN_POINT('Origin',(0.00264938241039218,0.0129,0.00511483151597876));
#48199=CARTESIAN_POINT('Origin',(0.00409095201815432,0.0129,0.00861244474036231));
#48200=CARTESIAN_POINT('Origin',(4.52079337441844E-5,0.0129,0.00735683187337397));
#48201=CARTESIAN_POINT('Origin',(-0.00968479566385333,0.0011,0.00433708631901139));
#48202=CARTESIAN_POINT('Origin',(4.5207933744215E-5,0.0011,0.00735683187337399));
#48203=CARTESIAN_POINT('Origin',(-0.000659221951814679,0.0011,0.00949866642219173));
#48204=CARTESIAN_POINT('Origin',(0.00264938241039218,0.0011,0.00511483151597876));
#48205=CARTESIAN_POINT('Origin',(0.00255021743138166,0.0129,0.00492053327615618));
#48206=CARTESIAN_POINT('Origin',(0.00257866842927369,0.0129,0.00497627854900125));
#48207=CARTESIAN_POINT('Origin',(5.18147787824767E-5,0.0129,0.00736000069289933));
#48208=CARTESIAN_POINT('Origin',(-0.00778675335060335,0.0129,0.00360041384088911));
#48209=CARTESIAN_POINT('Origin',(-0.00787324485361894,0.0298951219150416,
0.00378074470321196));
#48210=CARTESIAN_POINT('Origin',(-0.00787324485361894,0.0011,0.00378074470321196));
#48211=CARTESIAN_POINT('Origin',(-0.00787324485361894,0.0129,0.00378074470321196));
#48212=CARTESIAN_POINT('Origin',(-0.00922657982244437,0.0011,0.00290983456883857));
#48213=CARTESIAN_POINT('Origin',(-0.00778675335060335,0.0011,0.00360041384088911));
#48214=CARTESIAN_POINT('Origin',(-0.000670064127940984,0.0011,-0.00138910390576812));
#48215=CARTESIAN_POINT('Origin',(0.00257866842927369,0.0011,0.00497627854900125));
#48216=CARTESIAN_POINT('Origin',(0.00140969806589131,0.0129,0.00499913530392913));
#48217=CARTESIAN_POINT('Origin',(0.00139305626828132,0.0129,0.00499946069925261));
#48218=CARTESIAN_POINT('Origin',(-0.00787324485361894,0.0129,0.00378074470321196));
#48219=CARTESIAN_POINT('Origin',(-0.00804781744366059,0.0129,0.00368315161531047));
#48220=CARTESIAN_POINT('Origin',(-0.00787324485361894,0.0011,0.00378074470321196));
#48221=CARTESIAN_POINT('Origin',(-0.00804781744366059,0.0011,0.00368315161531047));
#48222=CARTESIAN_POINT('Origin',(-0.00922667024031924,0.0011,0.0052071070980081));
#48223=CARTESIAN_POINT('Origin',(0.00139305626828131,0.0011,0.00499946069925261));
#48224=CARTESIAN_POINT('Origin',(-0.0084990215765556,0.0129,0.00182721203634963));
#48225=CARTESIAN_POINT('Origin',(-0.00848709681638249,0.0129,0.00183103613732295));
#48226=CARTESIAN_POINT('Origin',(-0.00926982557395217,0.0129,0.003));
#48227=CARTESIAN_POINT('Origin',(-0.00853149850581388,0.0129,0.00181051559890248));
#48228=CARTESIAN_POINT('Origin',(-0.00926982557395217,0.0011,0.003));
#48229=CARTESIAN_POINT('Origin',(-0.00853149850581388,0.0011,0.00181051559890248));
#48230=CARTESIAN_POINT('Origin',(-0.00885692281820857,0.0011,0.001712438198831));
#48231=CARTESIAN_POINT('Origin',(-0.00848709681638249,0.0011,0.00183103613732295));
#48232=CARTESIAN_POINT('Origin',(-0.00842602321036556,0.0129,0.00164058925588855));
#48233=CARTESIAN_POINT('Origin',(-0.00842602321036556,0.0129,0.00164058925588855));
#48234=CARTESIAN_POINT('Origin',(-0.00842602321036556,0.0011,0.00164058925588855));
#48235=CARTESIAN_POINT('Origin',(-0.00842602321036556,0.0011,0.00164058925588855));
#48236=CARTESIAN_POINT('Origin',(-0.00842602321036556,0.0298951219150416,
0.00164058925588855));
#48237=CARTESIAN_POINT('Origin',(-0.00926982557395217,0.0011,0.003));
#48238=CARTESIAN_POINT('Origin',(-0.00926982557395217,0.0011,0.0036));
#48239=CARTESIAN_POINT('Origin',(-0.00926982557395217,0.0129,0.003));
#48240=CARTESIAN_POINT('Origin',(-0.00926982557395217,0.0129,0.0024));
#54555=UNCERTAINTY_MEASURE_WITH_UNIT(LENGTH_MEASURE(1.E-5),#54581,
'DISTANCE_ACCURACY_VALUE',
'Maximum model space distance between geometric entities at asserted c
onnectivities');
#54564=UNCERTAINTY_MEASURE_WITH_UNIT(LENGTH_MEASURE(1.E-5),#54581,
'DISTANCE_ACCURACY_VALUE',
'Maximum model space distance between geometric entities at asserted c
onnectivities');
#54571=(
GEOMETRIC_REPRESENTATION_CONTEXT(3)
GLOBAL_UNCERTAINTY_ASSIGNED_CONTEXT((#54555))
GLOBAL_UNIT_ASSIGNED_CONTEXT((#54581,#54582,#54583))
REPRESENTATION_CONTEXT('','3D')
);
#54580=(
GEOMETRIC_REPRESENTATION_CONTEXT(3)
GLOBAL_UNCERTAINTY_ASSIGNED_CONTEXT((#54564))
GLOBAL_UNIT_ASSIGNED_CONTEXT((#54581,#54582,#54583))
REPRESENTATION_CONTEXT('','3D')
);
#54581=(
LENGTH_UNIT()
NAMED_UNIT(*)
SI_UNIT($,.METRE.)
);
#54582=(
NAMED_UNIT(*)
PLANE_ANGLE_UNIT()
SI_UNIT($,.RADIAN.)
);
#54583=(
NAMED_UNIT(*)
SI_UNIT($,.STERADIAN.)
SOLID_ANGLE_UNIT()
);
#54590=SHAPE_DEFINITION_REPRESENTATION(#54605,#54635);
#54605=PRODUCT_DEFINITION_SHAPE('',$,#54651);
#54635=SHAPE_REPRESENTATION('',(#18812),#54571);
#54644=PRODUCT_DEFINITION_CONTEXT('part definition',#54691,'design');
#54651=PRODUCT_DEFINITION('Part_4','Part_4',#54666,#54644);
#54666=PRODUCT_DEFINITION_FORMATION('',$,#54699);
#54691=APPLICATION_CONTEXT(
'Core Data for Automotive Mechanical Design Process');
#54692=PRODUCT_CONTEXT('part definition',#54691,'mechanical');
#54699=PRODUCT('Part_4','Part_4','Part 1',(#54692));
#54716=PRESENTATION_STYLE_ASSIGNMENT((#54726));
#54726=SURFACE_STYLE_USAGE(.BOTH.,#54736);
#54736=SURFACE_SIDE_STYLE('',(#54746));
#54746=SURFACE_STYLE_FILL_AREA(#54756);
#54756=FILL_AREA_STYLE('Opaque(76,76,76)',(#54766));
#54766=FILL_AREA_STYLE_COLOUR('Opaque(76,76,76)',#54776);
#54776=COLOUR_RGB('Opaque(76,76,76)', 0.08235294, 0.09019608, 0.10196078);
ENDSEC;
END-ISO-10303-21;
